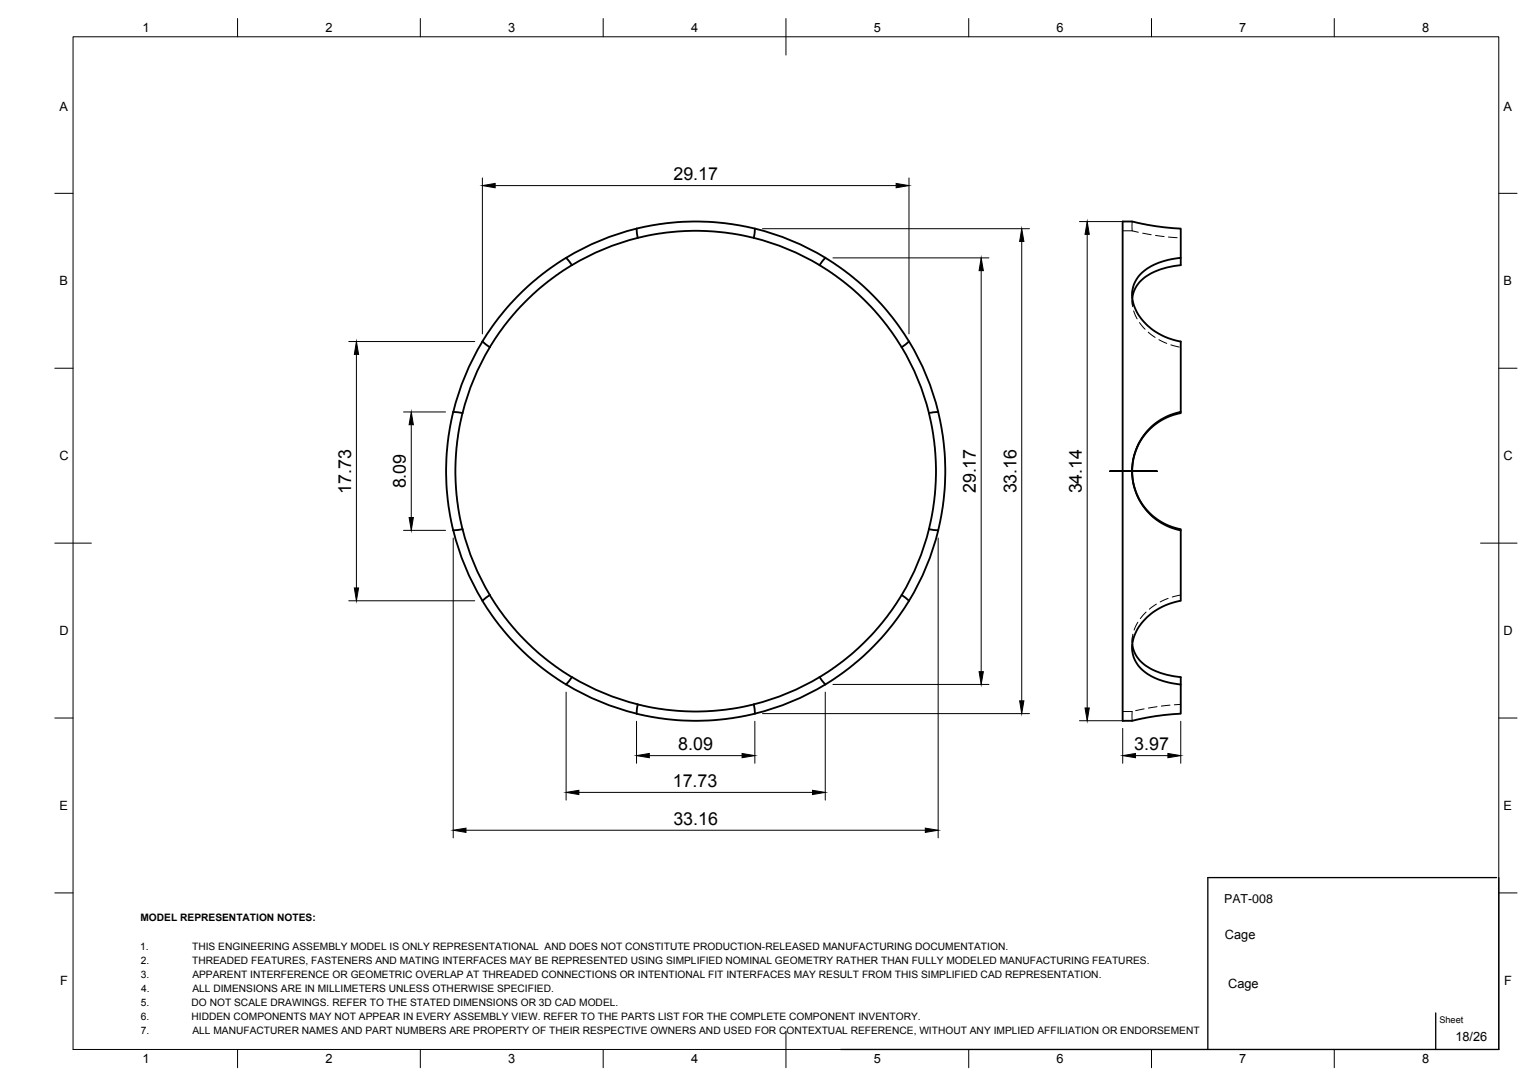
ISO-10303-21;
HEADER;
/* Generated by software containing ST-Developer
 * from STEP Tools, Inc. (www.steptools.com) 
 */

FILE_DESCRIPTION(
/* description */ ('Bearing housing with oil seal and end cap'),
/* implementation_level */ '2;1');

FILE_NAME(
/* name */ 'Cage.step',
/* time_stamp */ '2026-10-28T03:23:10-07:00',
/* author */ (''),
/* organization */ (''),
/* preprocessor_version */ 'ST-DEVELOPER v20.2',
/* originating_system */ 'Autodesk Translation Framework v15.17.0.0',
/* authorisation */ '');

FILE_SCHEMA (('AUTOMOTIVE_DESIGN { 1 0 10303 214 3 1 1 }'));
ENDSEC;

DATA;
#10=MECHANICAL_DESIGN_GEOMETRIC_PRESENTATION_REPRESENTATION('',(#277),#7871);
#159=B_SPLINE_CURVE_WITH_KNOTS('',3,(#6771,#6772,#6773,#6774,#6775,#6776,
#6777,#6778,#6779,#6780,#6781,#6782,#6783,#6784,#6785,#6786,#6787,#6788,
#6789,#6790,#6791,#6792),.UNSPECIFIED.,.F.,.F.,(4,2,2,2,2,2,2,2,2,2,4),
(0.0789094028588958,0.210573405340968,0.315860108011452,0.421146810681936,
0.522142632548711,0.623138454415485,0.72413427628226,0.825130098149035,
0.930416800819519,1.03570350349,1.16736750597208),.UNSPECIFIED.);
#160=B_SPLINE_CURVE_WITH_KNOTS('',3,(#6796,#6797,#6798,#6799,#6800,#6801,
#6802,#6803,#6804,#6805,#6806,#6807,#6808,#6809,#6810,#6811,#6812,#6813,
#6814,#6815,#6816,#6817),.UNSPECIFIED.,.F.,.F.,(4,2,2,2,2,2,2,2,2,2,4),
(0.0774793363974613,0.142088896491891,0.284177792983782,0.411119756996526,
0.514392970548519,0.617666184100513,0.720939397652506,0.8242126112045,0.951154575217244,
1.09324347170913,1.15785303180356),.UNSPECIFIED.);
#161=B_SPLINE_CURVE_WITH_KNOTS('',3,(#6823,#6824,#6825,#6826,#6827,#6828,
#6829,#6830,#6831,#6832,#6833,#6834,#6835,#6836,#6837,#6838,#6839,#6840,
#6841,#6842,#6843,#6844),.UNSPECIFIED.,.F.,.F.,(4,2,2,2,2,2,2,2,2,2,4),
(0.0774793363974613,0.142088896491891,0.284177792983782,0.411119756996525,
0.514392970548519,0.617666184100513,0.720939397652506,0.8242126112045,0.951154575217243,
1.09324347170913,1.15785303180356),.UNSPECIFIED.);
#162=B_SPLINE_CURVE_WITH_KNOTS('',3,(#6848,#6849,#6850,#6851,#6852,#6853,
#6854,#6855,#6856,#6857,#6858,#6859,#6860,#6861,#6862,#6863,#6864,#6865,
#6866,#6867,#6868,#6869),.UNSPECIFIED.,.F.,.F.,(4,2,2,2,2,2,2,2,2,2,4),
(0.0774793363974614,0.142088896491891,0.284177792983781,0.411119756996525,
0.514392970548519,0.617666184100512,0.720939397652506,0.824212611204499,
0.951154575217243,1.09324347170913,1.15785303180356),.UNSPECIFIED.);
#163=B_SPLINE_CURVE_WITH_KNOTS('',3,(#6873,#6874,#6875,#6876,#6877,#6878,
#6879,#6880,#6881,#6882,#6883,#6884),.UNSPECIFIED.,.F.,.F.,(4,2,2,2,2,4),
(0.0774793363974613,0.142088896491891,0.284177792983781,0.411119756996525,
0.514392970548519,0.617666184100512),.UNSPECIFIED.);
#164=B_SPLINE_CURVE_WITH_KNOTS('',3,(#6889,#6890,#6891,#6892,#6893,#6894,
#6895,#6896,#6897,#6898,#6899,#6900),.UNSPECIFIED.,.F.,.F.,(4,2,2,2,2,4),
(0.617666184100512,0.720939397652506,0.824212611204499,0.951154575217243,
1.09324347170913,1.15785303180356),.UNSPECIFIED.);
#165=B_SPLINE_CURVE_WITH_KNOTS('',3,(#6904,#6905,#6906,#6907,#6908,#6909,
#6910,#6911,#6912,#6913,#6914,#6915,#6916,#6917,#6918,#6919,#6920,#6921,
#6922,#6923,#6924,#6925),.UNSPECIFIED.,.F.,.F.,(4,2,2,2,2,2,2,2,2,2,4),
(0.0774793363974613,0.142088896491891,0.284177792983782,0.411119756996526,
0.514392970548519,0.617666184100513,0.720939397652507,0.8242126112045,0.951154575217245,
1.09324347170914,1.15785303180356),.UNSPECIFIED.);
#166=B_SPLINE_CURVE_WITH_KNOTS('',3,(#6929,#6930,#6931,#6932,#6933,#6934,
#6935,#6936,#6937,#6938,#6939,#6940,#6941,#6942,#6943,#6944,#6945,#6946,
#6947,#6948,#6949,#6950),.UNSPECIFIED.,.F.,.F.,(4,2,2,2,2,2,2,2,2,2,4),
(0.0774793363974613,0.142088896491891,0.284177792983782,0.411119756996526,
0.514392970548519,0.617666184100513,0.720939397652506,0.824212611204499,
0.951154575217243,1.09324347170913,1.15785303180356),.UNSPECIFIED.);
#167=B_SPLINE_CURVE_WITH_KNOTS('',3,(#6954,#6955,#6956,#6957,#6958,#6959,
#6960,#6961,#6962,#6963,#6964,#6965,#6966,#6967,#6968,#6969,#6970,#6971,
#6972,#6973,#6974,#6975),.UNSPECIFIED.,.F.,.F.,(4,2,2,2,2,2,2,2,2,2,4),
(0.0774793363974613,0.142088896491891,0.284177792983782,0.411119756996526,
0.514392970548519,0.617666184100513,0.720939397652506,0.8242126112045,0.951154575217244,
1.09324347170913,1.15785303180356),.UNSPECIFIED.);
#168=B_SPLINE_CURVE_WITH_KNOTS('',3,(#6979,#6980,#6981,#6982,#6983,#6984,
#6985,#6986,#6987,#6988,#6989,#6990,#6991,#6992,#6993,#6994,#6995,#6996,
#6997,#6998,#6999,#7000),.UNSPECIFIED.,.F.,.F.,(4,2,2,2,2,2,2,2,2,2,4),
(0.0774793363974613,0.142088896491891,0.284177792983782,0.411119756996526,
0.514392970548519,0.617666184100513,0.720939397652506,0.8242126112045,0.951154575217243,
1.09324347170913,1.15785303180356),.UNSPECIFIED.);
#169=B_SPLINE_CURVE_WITH_KNOTS('',3,(#7008,#7009,#7010,#7011,#7012,#7013,
#7014,#7015,#7016,#7017,#7018,#7019,#7020,#7021,#7022,#7023,#7024,#7025,
#7026,#7027,#7028,#7029),.UNSPECIFIED.,.F.,.F.,(4,2,2,2,2,2,2,2,2,2,4),
(0.0789094028588958,0.210573405340968,0.315860108011452,0.421146810681936,
0.522142632548711,0.623138454415485,0.72413427628226,0.825130098149035,
0.930416800819519,1.03570350349,1.16736750597208),.UNSPECIFIED.);
#170=B_SPLINE_CURVE_WITH_KNOTS('',3,(#7037,#7038,#7039,#7040,#7041,#7042,
#7043,#7044,#7045,#7046,#7047,#7048,#7049,#7050,#7051,#7052,#7053,#7054,
#7055,#7056,#7057,#7058),.UNSPECIFIED.,.F.,.F.,(4,2,2,2,2,2,2,2,2,2,4),
(0.0789094028588958,0.210573405340969,0.315860108011453,0.421146810681937,
0.522142632548712,0.623138454415486,0.724134276282261,0.825130098149035,
0.930416800819519,1.03570350349,1.16736750597208),.UNSPECIFIED.);
#171=B_SPLINE_CURVE_WITH_KNOTS('',3,(#7067,#7068,#7069,#7070,#7071,#7072,
#7073,#7074,#7075,#7076,#7077,#7078),.UNSPECIFIED.,.F.,.F.,(4,2,2,2,2,4),
(0.0789094028588958,0.210573405340968,0.315860108011452,0.421146810681937,
0.522142632548711,0.623138454415486),.UNSPECIFIED.);
#172=B_SPLINE_CURVE_WITH_KNOTS('',3,(#7080,#7081,#7082,#7083,#7084,#7085,
#7086,#7087,#7088,#7089,#7090,#7091),.UNSPECIFIED.,.F.,.F.,(4,2,2,2,2,4),
(0.623138454415486,0.72413427628226,0.825130098149035,0.930416800819519,
1.03570350349,1.16736750597208),.UNSPECIFIED.);
#173=B_SPLINE_CURVE_WITH_KNOTS('',3,(#7098,#7099,#7100,#7101,#7102,#7103,
#7104,#7105,#7106,#7107,#7108,#7109,#7110,#7111,#7112,#7113,#7114,#7115,
#7116,#7117,#7118,#7119),.UNSPECIFIED.,.F.,.F.,(4,2,2,2,2,2,2,2,2,2,4),
(0.0789094028588958,0.210573405340968,0.315860108011452,0.421146810681936,
0.522142632548711,0.623138454415486,0.72413427628226,0.825130098149035,
0.930416800819519,1.03570350349,1.16736750597208),.UNSPECIFIED.);
#174=B_SPLINE_CURVE_WITH_KNOTS('',3,(#7127,#7128,#7129,#7130,#7131,#7132,
#7133,#7134,#7135,#7136,#7137,#7138,#7139,#7140,#7141,#7142,#7143,#7144,
#7145,#7146,#7147,#7148),.UNSPECIFIED.,.F.,.F.,(4,2,2,2,2,2,2,2,2,2,4),
(0.0789094028588957,0.210573405340968,0.315860108011452,0.421146810681936,
0.522142632548711,0.623138454415485,0.72413427628226,0.825130098149035,
0.930416800819519,1.03570350349,1.16736750597207),.UNSPECIFIED.);
#175=B_SPLINE_CURVE_WITH_KNOTS('',3,(#7156,#7157,#7158,#7159,#7160,#7161,
#7162,#7163,#7164,#7165,#7166,#7167,#7168,#7169,#7170,#7171,#7172,#7173,
#7174,#7175,#7176,#7177),.UNSPECIFIED.,.F.,.F.,(4,2,2,2,2,2,2,2,2,2,4),
(0.0789094028588958,0.210573405340968,0.315860108011452,0.421146810681936,
0.522142632548711,0.623138454415486,0.72413427628226,0.825130098149035,
0.930416800819519,1.03570350349,1.16736750597208),.UNSPECIFIED.);
#176=B_SPLINE_CURVE_WITH_KNOTS('',3,(#7186,#7187,#7188,#7189,#7190,#7191,
#7192,#7193,#7194,#7195,#7196,#7197,#7198,#7199,#7200,#7201,#7202,#7203,
#7204,#7205,#7206,#7207),.UNSPECIFIED.,.F.,.F.,(4,2,2,2,2,2,2,2,2,2,4),
(0.0789094028588958,0.210573405340968,0.315860108011452,0.421146810681936,
0.522142632548711,0.623138454415485,0.72413427628226,0.825130098149035,
0.930416800819519,1.03570350349,1.16736750597208),.UNSPECIFIED.);
#193=SPHERICAL_SURFACE('',#4614,0.412776);
#194=SPHERICAL_SURFACE('',#4630,0.412776);
#195=SPHERICAL_SURFACE('',#4635,0.412776);
#196=SPHERICAL_SURFACE('',#4640,0.412776);
#197=SPHERICAL_SURFACE('',#4645,0.412776);
#198=SPHERICAL_SURFACE('',#4650,0.412776);
#199=SPHERICAL_SURFACE('',#4655,0.412776);
#200=SPHERICAL_SURFACE('',#4663,0.412776);
#228=SHAPE_REPRESENTATION_RELATIONSHIP('SRR','None',#7976,#249);
#249=ADVANCED_BREP_SHAPE_REPRESENTATION('',(#306),#7860);
#277=STYLED_ITEM('',(#8153),#306);
#306=MANIFOLD_SOLID_BREP('Continuous crown cage',#4103);
#378=FACE_BOUND('',#1013,.T.);
#475=PLANE('',#4627);
#476=PLANE('',#4632);
#477=PLANE('',#4637);
#478=PLANE('',#4642);
#479=PLANE('',#4647);
#480=PLANE('',#4652);
#481=PLANE('',#4661);
#482=PLANE('',#4665);
#483=PLANE('',#4666);
#681=FACE_OUTER_BOUND('',#995,.T.);
#682=FACE_OUTER_BOUND('',#996,.T.);
#683=FACE_OUTER_BOUND('',#997,.T.);
#684=FACE_OUTER_BOUND('',#998,.T.);
#685=FACE_OUTER_BOUND('',#999,.T.);
#686=FACE_OUTER_BOUND('',#1000,.T.);
#687=FACE_OUTER_BOUND('',#1001,.T.);
#688=FACE_OUTER_BOUND('',#1002,.T.);
#689=FACE_OUTER_BOUND('',#1003,.T.);
#690=FACE_OUTER_BOUND('',#1004,.T.);
#691=FACE_OUTER_BOUND('',#1005,.T.);
#692=FACE_OUTER_BOUND('',#1006,.T.);
#693=FACE_OUTER_BOUND('',#1007,.T.);
#694=FACE_OUTER_BOUND('',#1008,.T.);
#695=FACE_OUTER_BOUND('',#1009,.T.);
#696=FACE_OUTER_BOUND('',#1010,.T.);
#697=FACE_OUTER_BOUND('',#1011,.T.);
#698=FACE_OUTER_BOUND('',#1012,.T.);
#699=FACE_OUTER_BOUND('',#1014,.T.);
#995=EDGE_LOOP('',(#3235,#3236,#3237,#3238));
#996=EDGE_LOOP('',(#3239,#3240,#3241,#3242,#3243,#3244,#3245,#3246,#3247,
#3248,#3249,#3250,#3251,#3252,#3253,#3254,#3255,#3256,#3257,#3258));
#997=EDGE_LOOP('',(#3259,#3260,#3261,#3262));
#998=EDGE_LOOP('',(#3263,#3264,#3265,#3266));
#999=EDGE_LOOP('',(#3267,#3268,#3269,#3270));
#1000=EDGE_LOOP('',(#3271,#3272,#3273,#3274));
#1001=EDGE_LOOP('',(#3275,#3276,#3277,#3278));
#1002=EDGE_LOOP('',(#3279,#3280,#3281,#3282,#3283,#3284));
#1003=EDGE_LOOP('',(#3285,#3286,#3287,#3288));
#1004=EDGE_LOOP('',(#3289,#3290,#3291,#3292));
#1005=EDGE_LOOP('',(#3293,#3294,#3295,#3296));
#1006=EDGE_LOOP('',(#3297,#3298,#3299,#3300));
#1007=EDGE_LOOP('',(#3301,#3302,#3303,#3304));
#1008=EDGE_LOOP('',(#3305,#3306,#3307,#3308));
#1009=EDGE_LOOP('',(#3309,#3310,#3311,#3312,#3313,#3314,#3315,#3316,#3317,
#3318,#3319,#3320,#3321,#3322,#3323,#3324,#3325,#3326,#3327,#3328));
#1010=EDGE_LOOP('',(#3329,#3330,#3331,#3332));
#1011=EDGE_LOOP('',(#3333,#3334,#3335,#3336));
#1012=EDGE_LOOP('',(#3337));
#1013=EDGE_LOOP('',(#3338));
#1014=EDGE_LOOP('',(#3339,#3340,#3341,#3342));
#1271=LINE('',#6886,#1533);
#1272=LINE('',#7182,#1534);
#1533=VECTOR('',#5550,1.706752);
#1534=VECTOR('',#5627,1.643248);
#1793=CIRCLE('',#4615,0.405071403305639);
#1794=CIRCLE('',#4616,0.405071403305639);
#1795=CIRCLE('',#4618,1.706752);
#1796=CIRCLE('',#4619,1.706752);
#1797=CIRCLE('',#4620,1.706752);
#1798=CIRCLE('',#4621,1.706752);
#1799=CIRCLE('',#4622,1.706752);
#1800=CIRCLE('',#4623,1.706752);
#1801=CIRCLE('',#4624,1.706752);
#1802=CIRCLE('',#4625,1.706752);
#1803=CIRCLE('',#4626,1.706752);
#1804=CIRCLE('',#4628,1.643248);
#1805=CIRCLE('',#4629,0.405071403305639);
#1806=CIRCLE('',#4631,0.405071403305639);
#1807=CIRCLE('',#4633,1.643248);
#1808=CIRCLE('',#4634,0.405071403305639);
#1809=CIRCLE('',#4636,0.405071403305639);
#1810=CIRCLE('',#4638,1.643248);
#1811=CIRCLE('',#4639,0.405071403305639);
#1812=CIRCLE('',#4641,0.405071403305639);
#1813=CIRCLE('',#4643,1.643248);
#1814=CIRCLE('',#4644,0.405071403305639);
#1815=CIRCLE('',#4646,0.405071403305639);
#1816=CIRCLE('',#4648,1.643248);
#1817=CIRCLE('',#4649,0.405071403305639);
#1818=CIRCLE('',#4651,0.405071403305639);
#1819=CIRCLE('',#4653,1.643248);
#1820=CIRCLE('',#4654,0.405071403305639);
#1821=CIRCLE('',#4656,0.405071403305639);
#1822=CIRCLE('',#4658,1.643248);
#1823=CIRCLE('',#4659,1.643248);
#1824=CIRCLE('',#4660,1.643248);
#1825=CIRCLE('',#4662,0.405071403305639);
#1826=CIRCLE('',#4664,0.405071403305639);
#2063=VERTEX_POINT('',#6769);
#2064=VERTEX_POINT('',#6770);
#2065=VERTEX_POINT('',#6793);
#2066=VERTEX_POINT('',#6795);
#2067=VERTEX_POINT('',#6820);
#2068=VERTEX_POINT('',#6822);
#2069=VERTEX_POINT('',#6845);
#2070=VERTEX_POINT('',#6847);
#2071=VERTEX_POINT('',#6870);
#2072=VERTEX_POINT('',#6872);
#2073=VERTEX_POINT('',#6885);
#2074=VERTEX_POINT('',#6888);
#2075=VERTEX_POINT('',#6901);
#2076=VERTEX_POINT('',#6903);
#2077=VERTEX_POINT('',#6926);
#2078=VERTEX_POINT('',#6928);
#2079=VERTEX_POINT('',#6951);
#2080=VERTEX_POINT('',#6953);
#2081=VERTEX_POINT('',#6976);
#2082=VERTEX_POINT('',#6978);
#2083=VERTEX_POINT('',#7003);
#2084=VERTEX_POINT('',#7007);
#2085=VERTEX_POINT('',#7032);
#2086=VERTEX_POINT('',#7036);
#2087=VERTEX_POINT('',#7061);
#2088=VERTEX_POINT('',#7065);
#2089=VERTEX_POINT('',#7066);
#2090=VERTEX_POINT('',#7093);
#2091=VERTEX_POINT('',#7097);
#2092=VERTEX_POINT('',#7122);
#2093=VERTEX_POINT('',#7126);
#2094=VERTEX_POINT('',#7151);
#2095=VERTEX_POINT('',#7155);
#2096=VERTEX_POINT('',#7180);
#2097=VERTEX_POINT('',#7183);
#2098=VERTEX_POINT('',#7185);
#2481=EDGE_CURVE('',#2063,#2064,#159,.T.);
#2482=EDGE_CURVE('',#2065,#2063,#1793,.T.);
#2483=EDGE_CURVE('',#2066,#2065,#160,.T.);
#2484=EDGE_CURVE('',#2064,#2066,#1794,.T.);
#2485=EDGE_CURVE('',#2067,#2065,#1795,.T.);
#2486=EDGE_CURVE('',#2067,#2068,#161,.T.);
#2487=EDGE_CURVE('',#2069,#2068,#1796,.T.);
#2488=EDGE_CURVE('',#2069,#2070,#162,.T.);
#2489=EDGE_CURVE('',#2071,#2070,#1797,.T.);
#2490=EDGE_CURVE('',#2071,#2072,#163,.T.);
#2491=EDGE_CURVE('',#2072,#2073,#1271,.T.);
#2492=EDGE_CURVE('',#2073,#2073,#1798,.T.);
#2493=EDGE_CURVE('',#2072,#2074,#164,.T.);
#2494=EDGE_CURVE('',#2075,#2074,#1799,.T.);
#2495=EDGE_CURVE('',#2075,#2076,#165,.T.);
#2496=EDGE_CURVE('',#2077,#2076,#1800,.T.);
#2497=EDGE_CURVE('',#2077,#2078,#166,.T.);
#2498=EDGE_CURVE('',#2079,#2078,#1801,.T.);
#2499=EDGE_CURVE('',#2079,#2080,#167,.T.);
#2500=EDGE_CURVE('',#2081,#2080,#1802,.T.);
#2501=EDGE_CURVE('',#2081,#2082,#168,.T.);
#2502=EDGE_CURVE('',#2066,#2082,#1803,.T.);
#2503=EDGE_CURVE('',#2063,#2083,#1804,.T.);
#2504=EDGE_CURVE('',#2083,#2067,#1805,.T.);
#2505=EDGE_CURVE('',#2084,#2083,#169,.T.);
#2506=EDGE_CURVE('',#2068,#2084,#1806,.T.);
#2507=EDGE_CURVE('',#2084,#2085,#1807,.T.);
#2508=EDGE_CURVE('',#2085,#2069,#1808,.T.);
#2509=EDGE_CURVE('',#2086,#2085,#170,.T.);
#2510=EDGE_CURVE('',#2070,#2086,#1809,.T.);
#2511=EDGE_CURVE('',#2086,#2087,#1810,.T.);
#2512=EDGE_CURVE('',#2087,#2071,#1811,.T.);
#2513=EDGE_CURVE('',#2088,#2089,#171,.T.);
#2514=EDGE_CURVE('',#2074,#2088,#1812,.T.);
#2515=EDGE_CURVE('',#2089,#2087,#172,.T.);
#2516=EDGE_CURVE('',#2088,#2090,#1813,.T.);
#2517=EDGE_CURVE('',#2090,#2075,#1814,.T.);
#2518=EDGE_CURVE('',#2091,#2090,#173,.T.);
#2519=EDGE_CURVE('',#2076,#2091,#1815,.T.);
#2520=EDGE_CURVE('',#2091,#2092,#1816,.T.);
#2521=EDGE_CURVE('',#2092,#2077,#1817,.T.);
#2522=EDGE_CURVE('',#2093,#2092,#174,.T.);
#2523=EDGE_CURVE('',#2078,#2093,#1818,.T.);
#2524=EDGE_CURVE('',#2093,#2094,#1819,.T.);
#2525=EDGE_CURVE('',#2094,#2079,#1820,.T.);
#2526=EDGE_CURVE('',#2095,#2094,#175,.T.);
#2527=EDGE_CURVE('',#2080,#2095,#1821,.T.);
#2528=EDGE_CURVE('',#2096,#2096,#1822,.T.);
#2529=EDGE_CURVE('',#2096,#2089,#1272,.T.);
#2530=EDGE_CURVE('',#2097,#2064,#1823,.T.);
#2531=EDGE_CURVE('',#2097,#2098,#176,.T.);
#2532=EDGE_CURVE('',#2095,#2098,#1824,.T.);
#2533=EDGE_CURVE('',#2082,#2097,#1825,.T.);
#2534=EDGE_CURVE('',#2098,#2081,#1826,.T.);
#3235=ORIENTED_EDGE('',*,*,#2481,.F.);
#3236=ORIENTED_EDGE('',*,*,#2482,.F.);
#3237=ORIENTED_EDGE('',*,*,#2483,.F.);
#3238=ORIENTED_EDGE('',*,*,#2484,.F.);
#3239=ORIENTED_EDGE('',*,*,#2483,.T.);
#3240=ORIENTED_EDGE('',*,*,#2485,.F.);
#3241=ORIENTED_EDGE('',*,*,#2486,.T.);
#3242=ORIENTED_EDGE('',*,*,#2487,.F.);
#3243=ORIENTED_EDGE('',*,*,#2488,.T.);
#3244=ORIENTED_EDGE('',*,*,#2489,.F.);
#3245=ORIENTED_EDGE('',*,*,#2490,.T.);
#3246=ORIENTED_EDGE('',*,*,#2491,.T.);
#3247=ORIENTED_EDGE('',*,*,#2492,.F.);
#3248=ORIENTED_EDGE('',*,*,#2491,.F.);
#3249=ORIENTED_EDGE('',*,*,#2493,.T.);
#3250=ORIENTED_EDGE('',*,*,#2494,.F.);
#3251=ORIENTED_EDGE('',*,*,#2495,.T.);
#3252=ORIENTED_EDGE('',*,*,#2496,.F.);
#3253=ORIENTED_EDGE('',*,*,#2497,.T.);
#3254=ORIENTED_EDGE('',*,*,#2498,.F.);
#3255=ORIENTED_EDGE('',*,*,#2499,.T.);
#3256=ORIENTED_EDGE('',*,*,#2500,.F.);
#3257=ORIENTED_EDGE('',*,*,#2501,.T.);
#3258=ORIENTED_EDGE('',*,*,#2502,.F.);
#3259=ORIENTED_EDGE('',*,*,#2482,.T.);
#3260=ORIENTED_EDGE('',*,*,#2503,.T.);
#3261=ORIENTED_EDGE('',*,*,#2504,.T.);
#3262=ORIENTED_EDGE('',*,*,#2485,.T.);
#3263=ORIENTED_EDGE('',*,*,#2505,.F.);
#3264=ORIENTED_EDGE('',*,*,#2506,.F.);
#3265=ORIENTED_EDGE('',*,*,#2486,.F.);
#3266=ORIENTED_EDGE('',*,*,#2504,.F.);
#3267=ORIENTED_EDGE('',*,*,#2506,.T.);
#3268=ORIENTED_EDGE('',*,*,#2507,.T.);
#3269=ORIENTED_EDGE('',*,*,#2508,.T.);
#3270=ORIENTED_EDGE('',*,*,#2487,.T.);
#3271=ORIENTED_EDGE('',*,*,#2509,.F.);
#3272=ORIENTED_EDGE('',*,*,#2510,.F.);
#3273=ORIENTED_EDGE('',*,*,#2488,.F.);
#3274=ORIENTED_EDGE('',*,*,#2508,.F.);
#3275=ORIENTED_EDGE('',*,*,#2510,.T.);
#3276=ORIENTED_EDGE('',*,*,#2511,.T.);
#3277=ORIENTED_EDGE('',*,*,#2512,.T.);
#3278=ORIENTED_EDGE('',*,*,#2489,.T.);
#3279=ORIENTED_EDGE('',*,*,#2513,.F.);
#3280=ORIENTED_EDGE('',*,*,#2514,.F.);
#3281=ORIENTED_EDGE('',*,*,#2493,.F.);
#3282=ORIENTED_EDGE('',*,*,#2490,.F.);
#3283=ORIENTED_EDGE('',*,*,#2512,.F.);
#3284=ORIENTED_EDGE('',*,*,#2515,.F.);
#3285=ORIENTED_EDGE('',*,*,#2514,.T.);
#3286=ORIENTED_EDGE('',*,*,#2516,.T.);
#3287=ORIENTED_EDGE('',*,*,#2517,.T.);
#3288=ORIENTED_EDGE('',*,*,#2494,.T.);
#3289=ORIENTED_EDGE('',*,*,#2518,.F.);
#3290=ORIENTED_EDGE('',*,*,#2519,.F.);
#3291=ORIENTED_EDGE('',*,*,#2495,.F.);
#3292=ORIENTED_EDGE('',*,*,#2517,.F.);
#3293=ORIENTED_EDGE('',*,*,#2519,.T.);
#3294=ORIENTED_EDGE('',*,*,#2520,.T.);
#3295=ORIENTED_EDGE('',*,*,#2521,.T.);
#3296=ORIENTED_EDGE('',*,*,#2496,.T.);
#3297=ORIENTED_EDGE('',*,*,#2522,.F.);
#3298=ORIENTED_EDGE('',*,*,#2523,.F.);
#3299=ORIENTED_EDGE('',*,*,#2497,.F.);
#3300=ORIENTED_EDGE('',*,*,#2521,.F.);
#3301=ORIENTED_EDGE('',*,*,#2523,.T.);
#3302=ORIENTED_EDGE('',*,*,#2524,.T.);
#3303=ORIENTED_EDGE('',*,*,#2525,.T.);
#3304=ORIENTED_EDGE('',*,*,#2498,.T.);
#3305=ORIENTED_EDGE('',*,*,#2499,.F.);
#3306=ORIENTED_EDGE('',*,*,#2525,.F.);
#3307=ORIENTED_EDGE('',*,*,#2526,.F.);
#3308=ORIENTED_EDGE('',*,*,#2527,.F.);
#3309=ORIENTED_EDGE('',*,*,#2528,.F.);
#3310=ORIENTED_EDGE('',*,*,#2529,.T.);
#3311=ORIENTED_EDGE('',*,*,#2515,.T.);
#3312=ORIENTED_EDGE('',*,*,#2511,.F.);
#3313=ORIENTED_EDGE('',*,*,#2509,.T.);
#3314=ORIENTED_EDGE('',*,*,#2507,.F.);
#3315=ORIENTED_EDGE('',*,*,#2505,.T.);
#3316=ORIENTED_EDGE('',*,*,#2503,.F.);
#3317=ORIENTED_EDGE('',*,*,#2481,.T.);
#3318=ORIENTED_EDGE('',*,*,#2530,.F.);
#3319=ORIENTED_EDGE('',*,*,#2531,.T.);
#3320=ORIENTED_EDGE('',*,*,#2532,.F.);
#3321=ORIENTED_EDGE('',*,*,#2526,.T.);
#3322=ORIENTED_EDGE('',*,*,#2524,.F.);
#3323=ORIENTED_EDGE('',*,*,#2522,.T.);
#3324=ORIENTED_EDGE('',*,*,#2520,.F.);
#3325=ORIENTED_EDGE('',*,*,#2518,.T.);
#3326=ORIENTED_EDGE('',*,*,#2516,.F.);
#3327=ORIENTED_EDGE('',*,*,#2513,.T.);
#3328=ORIENTED_EDGE('',*,*,#2529,.F.);
#3329=ORIENTED_EDGE('',*,*,#2484,.T.);
#3330=ORIENTED_EDGE('',*,*,#2502,.T.);
#3331=ORIENTED_EDGE('',*,*,#2533,.T.);
#3332=ORIENTED_EDGE('',*,*,#2530,.T.);
#3333=ORIENTED_EDGE('',*,*,#2501,.F.);
#3334=ORIENTED_EDGE('',*,*,#2534,.F.);
#3335=ORIENTED_EDGE('',*,*,#2531,.F.);
#3336=ORIENTED_EDGE('',*,*,#2533,.F.);
#3337=ORIENTED_EDGE('',*,*,#2492,.T.);
#3338=ORIENTED_EDGE('',*,*,#2528,.T.);
#3339=ORIENTED_EDGE('',*,*,#2527,.T.);
#3340=ORIENTED_EDGE('',*,*,#2532,.T.);
#3341=ORIENTED_EDGE('',*,*,#2534,.T.);
#3342=ORIENTED_EDGE('',*,*,#2500,.T.);
#3807=CYLINDRICAL_SURFACE('',#4617,1.706752);
#3808=CYLINDRICAL_SURFACE('',#4657,1.643248);
#3963=ADVANCED_FACE('',(#681),#193,.F.);
#3964=ADVANCED_FACE('',(#682),#3807,.T.);
#3965=ADVANCED_FACE('',(#683),#475,.T.);
#3966=ADVANCED_FACE('',(#684),#194,.F.);
#3967=ADVANCED_FACE('',(#685),#476,.T.);
#3968=ADVANCED_FACE('',(#686),#195,.F.);
#3969=ADVANCED_FACE('',(#687),#477,.T.);
#3970=ADVANCED_FACE('',(#688),#196,.F.);
#3971=ADVANCED_FACE('',(#689),#478,.T.);
#3972=ADVANCED_FACE('',(#690),#197,.F.);
#3973=ADVANCED_FACE('',(#691),#479,.T.);
#3974=ADVANCED_FACE('',(#692),#198,.F.);
#3975=ADVANCED_FACE('',(#693),#480,.T.);
#3976=ADVANCED_FACE('',(#694),#199,.F.);
#3977=ADVANCED_FACE('',(#695),#3808,.F.);
#3978=ADVANCED_FACE('',(#696),#481,.T.);
#3979=ADVANCED_FACE('',(#697),#200,.F.);
#3980=ADVANCED_FACE('',(#698,#378),#482,.T.);
#3981=ADVANCED_FACE('',(#699),#483,.T.);
#4103=CLOSED_SHELL('',(#3963,#3964,#3965,#3966,#3967,#3968,#3969,#3970,
#3971,#3972,#3973,#3974,#3975,#3976,#3977,#3978,#3979,#3980,#3981));
#4613=AXIS2_PLACEMENT_3D('',#6767,#5534,#5535);
#4614=AXIS2_PLACEMENT_3D('',#6768,#5536,#5537);
#4615=AXIS2_PLACEMENT_3D('',#6794,#5538,#5539);
#4616=AXIS2_PLACEMENT_3D('',#6818,#5540,#5541);
#4617=AXIS2_PLACEMENT_3D('',#6819,#5542,#5543);
#4618=AXIS2_PLACEMENT_3D('',#6821,#5544,#5545);
#4619=AXIS2_PLACEMENT_3D('',#6846,#5546,#5547);
#4620=AXIS2_PLACEMENT_3D('',#6871,#5548,#5549);
#4621=AXIS2_PLACEMENT_3D('',#6887,#5551,#5552);
#4622=AXIS2_PLACEMENT_3D('',#6902,#5553,#5554);
#4623=AXIS2_PLACEMENT_3D('',#6927,#5555,#5556);
#4624=AXIS2_PLACEMENT_3D('',#6952,#5557,#5558);
#4625=AXIS2_PLACEMENT_3D('',#6977,#5559,#5560);
#4626=AXIS2_PLACEMENT_3D('',#7001,#5561,#5562);
#4627=AXIS2_PLACEMENT_3D('',#7002,#5563,#5564);
#4628=AXIS2_PLACEMENT_3D('',#7004,#5565,#5566);
#4629=AXIS2_PLACEMENT_3D('',#7005,#5567,#5568);
#4630=AXIS2_PLACEMENT_3D('',#7006,#5569,#5570);
#4631=AXIS2_PLACEMENT_3D('',#7030,#5571,#5572);
#4632=AXIS2_PLACEMENT_3D('',#7031,#5573,#5574);
#4633=AXIS2_PLACEMENT_3D('',#7033,#5575,#5576);
#4634=AXIS2_PLACEMENT_3D('',#7034,#5577,#5578);
#4635=AXIS2_PLACEMENT_3D('',#7035,#5579,#5580);
#4636=AXIS2_PLACEMENT_3D('',#7059,#5581,#5582);
#4637=AXIS2_PLACEMENT_3D('',#7060,#5583,#5584);
#4638=AXIS2_PLACEMENT_3D('',#7062,#5585,#5586);
#4639=AXIS2_PLACEMENT_3D('',#7063,#5587,#5588);
#4640=AXIS2_PLACEMENT_3D('',#7064,#5589,#5590);
#4641=AXIS2_PLACEMENT_3D('',#7079,#5591,#5592);
#4642=AXIS2_PLACEMENT_3D('',#7092,#5593,#5594);
#4643=AXIS2_PLACEMENT_3D('',#7094,#5595,#5596);
#4644=AXIS2_PLACEMENT_3D('',#7095,#5597,#5598);
#4645=AXIS2_PLACEMENT_3D('',#7096,#5599,#5600);
#4646=AXIS2_PLACEMENT_3D('',#7120,#5601,#5602);
#4647=AXIS2_PLACEMENT_3D('',#7121,#5603,#5604);
#4648=AXIS2_PLACEMENT_3D('',#7123,#5605,#5606);
#4649=AXIS2_PLACEMENT_3D('',#7124,#5607,#5608);
#4650=AXIS2_PLACEMENT_3D('',#7125,#5609,#5610);
#4651=AXIS2_PLACEMENT_3D('',#7149,#5611,#5612);
#4652=AXIS2_PLACEMENT_3D('',#7150,#5613,#5614);
#4653=AXIS2_PLACEMENT_3D('',#7152,#5615,#5616);
#4654=AXIS2_PLACEMENT_3D('',#7153,#5617,#5618);
#4655=AXIS2_PLACEMENT_3D('',#7154,#5619,#5620);
#4656=AXIS2_PLACEMENT_3D('',#7178,#5621,#5622);
#4657=AXIS2_PLACEMENT_3D('',#7179,#5623,#5624);
#4658=AXIS2_PLACEMENT_3D('',#7181,#5625,#5626);
#4659=AXIS2_PLACEMENT_3D('',#7184,#5628,#5629);
#4660=AXIS2_PLACEMENT_3D('',#7208,#5630,#5631);
#4661=AXIS2_PLACEMENT_3D('',#7209,#5632,#5633);
#4662=AXIS2_PLACEMENT_3D('',#7210,#5634,#5635);
#4663=AXIS2_PLACEMENT_3D('',#7211,#5636,#5637);
#4664=AXIS2_PLACEMENT_3D('',#7212,#5638,#5639);
#4665=AXIS2_PLACEMENT_3D('',#7213,#5640,#5641);
#4666=AXIS2_PLACEMENT_3D('',#7214,#5642,#5643);
#5534=DIRECTION('axis',(0.,0.,1.));
#5535=DIRECTION('refdir',(1.,0.,0.));
#5536=DIRECTION('center_axis',(0.,0.,1.));
#5537=DIRECTION('ref_axis',(1.,0.,0.));
#5538=DIRECTION('center_axis',(0.,-1.,0.));
#5539=DIRECTION('ref_axis',(0.,0.,-1.));
#5540=DIRECTION('center_axis',(0.,-1.,0.));
#5541=DIRECTION('ref_axis',(0.,0.,-1.));
#5542=DIRECTION('center_axis',(0.,1.,0.));
#5543=DIRECTION('ref_axis',(1.,0.,0.));
#5544=DIRECTION('center_axis',(0.,1.,0.));
#5545=DIRECTION('ref_axis',(1.,0.,0.));
#5546=DIRECTION('center_axis',(0.,1.,0.));
#5547=DIRECTION('ref_axis',(1.,0.,0.));
#5548=DIRECTION('center_axis',(0.,1.,0.));
#5549=DIRECTION('ref_axis',(1.,0.,0.));
#5550=DIRECTION('',(0.,-1.,0.));
#5551=DIRECTION('center_axis',(0.,-1.,0.));
#5552=DIRECTION('ref_axis',(1.,0.,0.));
#5553=DIRECTION('center_axis',(0.,1.,0.));
#5554=DIRECTION('ref_axis',(1.,0.,0.));
#5555=DIRECTION('center_axis',(0.,1.,0.));
#5556=DIRECTION('ref_axis',(1.,0.,0.));
#5557=DIRECTION('center_axis',(0.,1.,0.));
#5558=DIRECTION('ref_axis',(1.,0.,0.));
#5559=DIRECTION('center_axis',(0.,1.,0.));
#5560=DIRECTION('ref_axis',(1.,0.,0.));
#5561=DIRECTION('center_axis',(0.,1.,0.));
#5562=DIRECTION('ref_axis',(1.,0.,0.));
#5563=DIRECTION('center_axis',(0.,1.,0.));
#5564=DIRECTION('ref_axis',(1.,0.,0.));
#5565=DIRECTION('center_axis',(0.,-1.,0.));
#5566=DIRECTION('ref_axis',(1.,0.,0.));
#5567=DIRECTION('center_axis',(0.,-1.,0.));
#5568=DIRECTION('ref_axis',(0.,0.,-1.));
#5569=DIRECTION('center_axis',(6.12323399573677E-17,0.,1.));
#5570=DIRECTION('ref_axis',(1.,0.,0.));
#5571=DIRECTION('center_axis',(0.,-1.,0.));
#5572=DIRECTION('ref_axis',(0.,0.,-1.));
#5573=DIRECTION('center_axis',(0.,1.,0.));
#5574=DIRECTION('ref_axis',(1.,0.,0.));
#5575=DIRECTION('center_axis',(0.,-1.,0.));
#5576=DIRECTION('ref_axis',(1.,0.,0.));
#5577=DIRECTION('center_axis',(0.,-1.,0.));
#5578=DIRECTION('ref_axis',(0.,0.,-1.));
#5579=DIRECTION('center_axis',(0.,0.,1.));
#5580=DIRECTION('ref_axis',(1.,0.,0.));
#5581=DIRECTION('center_axis',(0.,-1.,0.));
#5582=DIRECTION('ref_axis',(0.,0.,-1.));
#5583=DIRECTION('center_axis',(0.,1.,0.));
#5584=DIRECTION('ref_axis',(1.,0.,0.));
#5585=DIRECTION('center_axis',(0.,-1.,0.));
#5586=DIRECTION('ref_axis',(1.,0.,0.));
#5587=DIRECTION('center_axis',(0.,-1.,0.));
#5588=DIRECTION('ref_axis',(0.,0.,-1.));
#5589=DIRECTION('center_axis',(0.,0.,1.));
#5590=DIRECTION('ref_axis',(1.,0.,0.));
#5591=DIRECTION('center_axis',(0.,-1.,0.));
#5592=DIRECTION('ref_axis',(0.,0.,-1.));
#5593=DIRECTION('center_axis',(0.,1.,0.));
#5594=DIRECTION('ref_axis',(1.,0.,0.));
#5595=DIRECTION('center_axis',(0.,-1.,0.));
#5596=DIRECTION('ref_axis',(1.,0.,0.));
#5597=DIRECTION('center_axis',(0.,-1.,0.));
#5598=DIRECTION('ref_axis',(0.,0.,-1.));
#5599=DIRECTION('center_axis',(0.,0.,1.));
#5600=DIRECTION('ref_axis',(1.,0.,0.));
#5601=DIRECTION('center_axis',(0.,-1.,0.));
#5602=DIRECTION('ref_axis',(0.,0.,-1.));
#5603=DIRECTION('center_axis',(0.,1.,0.));
#5604=DIRECTION('ref_axis',(1.,0.,0.));
#5605=DIRECTION('center_axis',(0.,-1.,0.));
#5606=DIRECTION('ref_axis',(1.,0.,0.));
#5607=DIRECTION('center_axis',(0.,-1.,0.));
#5608=DIRECTION('ref_axis',(0.,0.,-1.));
#5609=DIRECTION('center_axis',(6.12323399573676E-17,0.,1.));
#5610=DIRECTION('ref_axis',(1.,0.,0.));
#5611=DIRECTION('center_axis',(0.,-1.,0.));
#5612=DIRECTION('ref_axis',(0.,0.,-1.));
#5613=DIRECTION('center_axis',(0.,1.,0.));
#5614=DIRECTION('ref_axis',(1.,0.,0.));
#5615=DIRECTION('center_axis',(0.,-1.,0.));
#5616=DIRECTION('ref_axis',(1.,0.,0.));
#5617=DIRECTION('center_axis',(0.,-1.,0.));
#5618=DIRECTION('ref_axis',(0.,0.,-1.));
#5619=DIRECTION('center_axis',(0.,0.,1.));
#5620=DIRECTION('ref_axis',(1.,0.,0.));
#5621=DIRECTION('center_axis',(0.,-1.,0.));
#5622=DIRECTION('ref_axis',(0.,0.,-1.));
#5623=DIRECTION('center_axis',(0.,1.,0.));
#5624=DIRECTION('ref_axis',(1.,0.,0.));
#5625=DIRECTION('center_axis',(0.,1.,0.));
#5626=DIRECTION('ref_axis',(1.,0.,0.));
#5627=DIRECTION('',(0.,1.,0.));
#5628=DIRECTION('center_axis',(0.,-1.,0.));
#5629=DIRECTION('ref_axis',(1.,0.,0.));
#5630=DIRECTION('center_axis',(0.,-1.,0.));
#5631=DIRECTION('ref_axis',(1.,0.,0.));
#5632=DIRECTION('center_axis',(0.,1.,0.));
#5633=DIRECTION('ref_axis',(1.,0.,0.));
#5634=DIRECTION('center_axis',(0.,-1.,0.));
#5635=DIRECTION('ref_axis',(0.,0.,-1.));
#5636=DIRECTION('center_axis',(0.,0.,1.));
#5637=DIRECTION('ref_axis',(1.,0.,0.));
#5638=DIRECTION('center_axis',(0.,-1.,0.));
#5639=DIRECTION('ref_axis',(0.,0.,-1.));
#5640=DIRECTION('center_axis',(0.,-1.,0.));
#5641=DIRECTION('ref_axis',(-1.,0.,0.));
#5642=DIRECTION('center_axis',(0.,1.,0.));
#5643=DIRECTION('ref_axis',(1.,0.,0.));
#6767=CARTESIAN_POINT('',(0.,0.,0.));
#6768=CARTESIAN_POINT('Origin',(1.18440385848747,0.,1.18440385848747));
#6769=CARTESIAN_POINT('',(0.846804978391753,-0.07938,1.40825612658882));
#6770=CARTESIAN_POINT('',(1.40825612658882,-0.07938,0.846804978391754));
#6771=CARTESIAN_POINT('Ctrl Pts',(0.846804978391752,-0.0793800000000001,
1.40825612658882));
#6772=CARTESIAN_POINT('Ctrl Pts',(0.854205272175554,-0.123401821157026,
1.40380622184538));
#6773=CARTESIAN_POINT('Ctrl Pts',(0.867957148219441,-0.166543350814306,
1.39550172959303));
#6774=CARTESIAN_POINT('Ctrl Pts',(0.902193646979982,-0.237231147975234,
1.3735491215176));
#6775=CARTESIAN_POINT('Ctrl Pts',(0.920778333482564,-0.266264900654909,
1.36127834356734));
#6776=CARTESIAN_POINT('Ctrl Pts',(0.962485392528369,-0.317195968905306,
1.33211611256184));
#6777=CARTESIAN_POINT('Ctrl Pts',(0.985600426557816,-0.33909093068465,1.31521005565926));
#6778=CARTESIAN_POINT('Ctrl Pts',(1.03253285680459,-0.373586846396559,1.27866649102984));
#6779=CARTESIAN_POINT('Ctrl Pts',(1.05871835910697,-0.388086240756494,1.25722555095714));
#6780=CARTESIAN_POINT('Ctrl Pts',(1.11153475808518,-0.407068917407805,1.2107812086231));
#6781=CARTESIAN_POINT('Ctrl Pts',(1.13814686046673,-0.411552957311693,1.18575674747573));
#6782=CARTESIAN_POINT('Ctrl Pts',(1.18575674747573,-0.411552957311693,1.13814686046673));
#6783=CARTESIAN_POINT('Ctrl Pts',(1.2107812086231,-0.407068917407805,1.11153475808518));
#6784=CARTESIAN_POINT('Ctrl Pts',(1.25722555095713,-0.388086240756494,1.05871835910697));
#6785=CARTESIAN_POINT('Ctrl Pts',(1.27866649102984,-0.373586846396559,1.03253285680459));
#6786=CARTESIAN_POINT('Ctrl Pts',(1.31521005565926,-0.33909093068465,0.985600426557816));
#6787=CARTESIAN_POINT('Ctrl Pts',(1.33211611256184,-0.317195968905306,0.962485392528369));
#6788=CARTESIAN_POINT('Ctrl Pts',(1.36127834356734,-0.266264900654909,0.920778333482565));
#6789=CARTESIAN_POINT('Ctrl Pts',(1.3735491215176,-0.237231147975234,0.902193646979983));
#6790=CARTESIAN_POINT('Ctrl Pts',(1.39550172959303,-0.166543350814306,0.867957148219442));
#6791=CARTESIAN_POINT('Ctrl Pts',(1.40380622184538,-0.123401821157026,0.854205272175555));
#6792=CARTESIAN_POINT('Ctrl Pts',(1.40825612658882,-0.0793800000000001,
0.846804978391753));
#6793=CARTESIAN_POINT('',(0.886256117232623,-0.07938,1.45861320581289));
#6794=CARTESIAN_POINT('Origin',(1.18440385848747,-0.07938,1.18440385848747));
#6795=CARTESIAN_POINT('',(1.45861320581289,-0.07938,0.886256117232624));
#6796=CARTESIAN_POINT('Ctrl Pts',(1.45861320581289,-0.0793800000000001,
0.886256117232623));
#6797=CARTESIAN_POINT('Ctrl Pts',(1.45630208793976,-0.101649918886749,0.890059788636852));
#6798=CARTESIAN_POINT('Ctrl Pts',(1.45296717977858,-0.123823518623746,0.895520212222107));
#6799=CARTESIAN_POINT('Ctrl Pts',(1.43904931717599,-0.192480977588836,0.917859913453975));
#6800=CARTESIAN_POINT('Ctrl Pts',(1.4243271592157,-0.236152929235938,0.940896403863072));
#6801=CARTESIAN_POINT('Ctrl Pts',(1.39055359345152,-0.303141259068212,0.990027513266106));
#6802=CARTESIAN_POINT('Ctrl Pts',(1.36743459453896,-0.335108247315849,1.02199477007745));
#6803=CARTESIAN_POINT('Ctrl Pts',(1.32643091652006,-0.373243761060364,1.07446535104584));
#6804=CARTESIAN_POINT('Ctrl Pts',(1.30441816675528,-0.387888272594439,1.10126842659597));
#6805=CARTESIAN_POINT('Ctrl Pts',(1.25681160160691,-0.407041111792943,1.15530234155453));
#6806=CARTESIAN_POINT('Ctrl Pts',(1.23119764287622,-0.411552957311693,1.18251418313119));
#6807=CARTESIAN_POINT('Ctrl Pts',(1.18251418313119,-0.411552957311693,1.23119764287622));
#6808=CARTESIAN_POINT('Ctrl Pts',(1.15530234155453,-0.407041111792943,1.25681160160691));
#6809=CARTESIAN_POINT('Ctrl Pts',(1.10126842659597,-0.387888272594439,1.30441816675528));
#6810=CARTESIAN_POINT('Ctrl Pts',(1.07446535104584,-0.373243761060364,1.32643091652006));
#6811=CARTESIAN_POINT('Ctrl Pts',(1.02199477007745,-0.335108247315848,1.36743459453896));
#6812=CARTESIAN_POINT('Ctrl Pts',(0.990027513266105,-0.303141259068211,
1.39055359345152));
#6813=CARTESIAN_POINT('Ctrl Pts',(0.940896403863071,-0.236152929235937,
1.42432715921571));
#6814=CARTESIAN_POINT('Ctrl Pts',(0.917859913453974,-0.192480977588835,
1.43904931717599));
#6815=CARTESIAN_POINT('Ctrl Pts',(0.895520212222106,-0.123823518623745,
1.45296717977858));
#6816=CARTESIAN_POINT('Ctrl Pts',(0.890059788636851,-0.101649918886749,
1.45630208793976));
#6817=CARTESIAN_POINT('Ctrl Pts',(0.886256117232622,-0.0793800000000001,
1.45861320581289));
#6818=CARTESIAN_POINT('Origin',(1.18440385848747,-0.07938,1.18440385848747));
#6819=CARTESIAN_POINT('Origin',(0.,-0.27783,0.));
#6820=CARTESIAN_POINT('',(0.404717578595295,-0.07938,1.65807299932179));
#6821=CARTESIAN_POINT('Origin',(0.,-0.07938,0.));
#6822=CARTESIAN_POINT('',(-0.404717578595296,-0.07938,1.65807299932179));
#6823=CARTESIAN_POINT('Ctrl Pts',(0.404717578595296,-0.0793800000000001,
1.65807299932179));
#6824=CARTESIAN_POINT('Ctrl Pts',(0.400393769631747,-0.101649918886749,
1.65912839404491));
#6825=CARTESIAN_POINT('Ctrl Pts',(0.394174530911058,-0.123823518623745,
1.66063136041479));
#6826=CARTESIAN_POINT('Ctrl Pts',(0.368536561654407,-0.192480977588835,
1.66658649961961));
#6827=CARTESIAN_POINT('Ctrl Pts',(0.341837165343982,-0.236152929235937,
1.67246562047521));
#6828=CARTESIAN_POINT('Ctrl Pts',(0.283214707341173,-0.303141259068211,
1.68332504372461));
#6829=CARTESIAN_POINT('Ctrl Pts',(0.244262842368623,-0.335108247315849,
1.68958170688653));
#6830=CARTESIAN_POINT('Ctrl Pts',(0.178166559972324,-0.373243761060364,
1.69769003172132));
#6831=CARTESIAN_POINT('Ctrl Pts',(0.143648558862931,-0.387888272594439,
1.70107730356824));
#6832=CARTESIAN_POINT('Ctrl Pts',(0.0717778861362652,-0.407041111792943,
1.70562212620408));
#6833=CARTESIAN_POINT('Ctrl Pts',(0.0344244045173309,-0.411552957311693,
1.706752));
#6834=CARTESIAN_POINT('Ctrl Pts',(-0.0344244045173315,-0.411552957311693,
1.706752));
#6835=CARTESIAN_POINT('Ctrl Pts',(-0.0717778861362658,-0.407041111792943,
1.70562212620408));
#6836=CARTESIAN_POINT('Ctrl Pts',(-0.143648558862932,-0.387888272594439,
1.70107730356824));
#6837=CARTESIAN_POINT('Ctrl Pts',(-0.178166559972325,-0.373243761060364,
1.69769003172132));
#6838=CARTESIAN_POINT('Ctrl Pts',(-0.244262842368624,-0.335108247315849,
1.68958170688653));
#6839=CARTESIAN_POINT('Ctrl Pts',(-0.283214707341173,-0.303141259068212,
1.68332504372461));
#6840=CARTESIAN_POINT('Ctrl Pts',(-0.341837165343982,-0.236152929235937,
1.67246562047521));
#6841=CARTESIAN_POINT('Ctrl Pts',(-0.368536561654408,-0.192480977588835,
1.66658649961961));
#6842=CARTESIAN_POINT('Ctrl Pts',(-0.394174530911059,-0.123823518623745,
1.66063136041479));
#6843=CARTESIAN_POINT('Ctrl Pts',(-0.400393769631748,-0.101649918886749,
1.65912839404491));
#6844=CARTESIAN_POINT('Ctrl Pts',(-0.404717578595297,-0.0793800000000001,
1.65807299932179));
#6845=CARTESIAN_POINT('',(-0.886256117232624,-0.07938,1.45861320581289));
#6846=CARTESIAN_POINT('Origin',(0.,-0.07938,0.));
#6847=CARTESIAN_POINT('',(-1.45861320581289,-0.07938,0.886256117232623));
#6848=CARTESIAN_POINT('Ctrl Pts',(-0.886256117232623,-0.0793800000000001,
1.45861320581289));
#6849=CARTESIAN_POINT('Ctrl Pts',(-0.890059788636852,-0.101649918886749,
1.45630208793976));
#6850=CARTESIAN_POINT('Ctrl Pts',(-0.895520212222106,-0.123823518623745,
1.45296717977858));
#6851=CARTESIAN_POINT('Ctrl Pts',(-0.917859913453974,-0.192480977588835,
1.43904931717599));
#6852=CARTESIAN_POINT('Ctrl Pts',(-0.940896403863071,-0.236152929235937,
1.4243271592157));
#6853=CARTESIAN_POINT('Ctrl Pts',(-0.990027513266105,-0.303141259068211,
1.39055359345152));
#6854=CARTESIAN_POINT('Ctrl Pts',(-1.02199477007745,-0.335108247315848,
1.36743459453896));
#6855=CARTESIAN_POINT('Ctrl Pts',(-1.07446535104584,-0.373243761060364,
1.32643091652006));
#6856=CARTESIAN_POINT('Ctrl Pts',(-1.10126842659597,-0.387888272594439,
1.30441816675528));
#6857=CARTESIAN_POINT('Ctrl Pts',(-1.15530234155453,-0.407041111792943,
1.25681160160691));
#6858=CARTESIAN_POINT('Ctrl Pts',(-1.18251418313119,-0.411552957311693,
1.23119764287622));
#6859=CARTESIAN_POINT('Ctrl Pts',(-1.23119764287622,-0.411552957311693,
1.18251418313119));
#6860=CARTESIAN_POINT('Ctrl Pts',(-1.25681160160691,-0.407041111792943,
1.15530234155453));
#6861=CARTESIAN_POINT('Ctrl Pts',(-1.30441816675528,-0.387888272594439,
1.10126842659597));
#6862=CARTESIAN_POINT('Ctrl Pts',(-1.32643091652006,-0.373243761060365,
1.07446535104584));
#6863=CARTESIAN_POINT('Ctrl Pts',(-1.36743459453896,-0.335108247315849,
1.02199477007745));
#6864=CARTESIAN_POINT('Ctrl Pts',(-1.39055359345152,-0.303141259068212,
0.990027513266106));
#6865=CARTESIAN_POINT('Ctrl Pts',(-1.4243271592157,-0.236152929235938,0.940896403863071));
#6866=CARTESIAN_POINT('Ctrl Pts',(-1.43904931717599,-0.192480977588836,
0.917859913453974));
#6867=CARTESIAN_POINT('Ctrl Pts',(-1.45296717977858,-0.123823518623746,
0.895520212222106));
#6868=CARTESIAN_POINT('Ctrl Pts',(-1.45630208793976,-0.101649918886749,
0.890059788636852));
#6869=CARTESIAN_POINT('Ctrl Pts',(-1.45861320581289,-0.0793800000000001,
0.886256117232623));
#6870=CARTESIAN_POINT('',(-1.65807299932179,-0.07938,0.404717578595295));
#6871=CARTESIAN_POINT('Origin',(0.,-0.07938,0.));
#6872=CARTESIAN_POINT('',(-1.706752,-0.411552957311693,2.08591827245526E-16));
#6873=CARTESIAN_POINT('Ctrl Pts',(-1.65807299932179,-0.0793800000000001,
0.404717578595296));
#6874=CARTESIAN_POINT('Ctrl Pts',(-1.65912839404491,-0.101649918886749,
0.400393769631747));
#6875=CARTESIAN_POINT('Ctrl Pts',(-1.66063136041479,-0.123823518623745,
0.394174530911058));
#6876=CARTESIAN_POINT('Ctrl Pts',(-1.66658649961961,-0.192480977588835,
0.368536561654407));
#6877=CARTESIAN_POINT('Ctrl Pts',(-1.67246562047521,-0.236152929235937,
0.341837165343982));
#6878=CARTESIAN_POINT('Ctrl Pts',(-1.68332504372461,-0.303141259068211,
0.283214707341173));
#6879=CARTESIAN_POINT('Ctrl Pts',(-1.68958170688653,-0.335108247315848,
0.244262842368623));
#6880=CARTESIAN_POINT('Ctrl Pts',(-1.69769003172132,-0.373243761060364,
0.178166559972324));
#6881=CARTESIAN_POINT('Ctrl Pts',(-1.70107730356824,-0.387888272594439,
0.143648558862931));
#6882=CARTESIAN_POINT('Ctrl Pts',(-1.70562212620408,-0.407041111792943,
0.0717778861362656));
#6883=CARTESIAN_POINT('Ctrl Pts',(-1.706752,-0.411552957311693,0.0344244045173313));
#6884=CARTESIAN_POINT('Ctrl Pts',(-1.706752,-0.411552957311693,2.08166817117217E-16));
#6885=CARTESIAN_POINT('',(-1.706752,-0.47628,2.09016837373834E-16));
#6886=CARTESIAN_POINT('',(-1.706752,-0.27783,2.09016837373834E-16));
#6887=CARTESIAN_POINT('Origin',(0.,-0.47628,0.));
#6888=CARTESIAN_POINT('',(-1.65807299932179,-0.07938,-0.404717578595296));
#6889=CARTESIAN_POINT('Ctrl Pts',(-1.706752,-0.411552957311693,2.0122792321331E-16));
#6890=CARTESIAN_POINT('Ctrl Pts',(-1.706752,-0.411552957311693,-0.0344244045173309));
#6891=CARTESIAN_POINT('Ctrl Pts',(-1.70562212620408,-0.407041111792943,
-0.0717778861362652));
#6892=CARTESIAN_POINT('Ctrl Pts',(-1.70107730356824,-0.387888272594439,
-0.143648558862931));
#6893=CARTESIAN_POINT('Ctrl Pts',(-1.69769003172132,-0.373243761060365,
-0.178166559972324));
#6894=CARTESIAN_POINT('Ctrl Pts',(-1.68958170688653,-0.335108247315849,
-0.244262842368623));
#6895=CARTESIAN_POINT('Ctrl Pts',(-1.68332504372461,-0.303141259068212,
-0.283214707341173));
#6896=CARTESIAN_POINT('Ctrl Pts',(-1.67246562047521,-0.236152929235938,
-0.341837165343982));
#6897=CARTESIAN_POINT('Ctrl Pts',(-1.66658649961961,-0.192480977588836,
-0.368536561654407));
#6898=CARTESIAN_POINT('Ctrl Pts',(-1.66063136041479,-0.123823518623745,
-0.394174530911059));
#6899=CARTESIAN_POINT('Ctrl Pts',(-1.65912839404491,-0.101649918886749,
-0.400393769631748));
#6900=CARTESIAN_POINT('Ctrl Pts',(-1.65807299932179,-0.0793800000000001,
-0.404717578595296));
#6901=CARTESIAN_POINT('',(-1.45861320581289,-0.07938,-0.886256117232623));
#6902=CARTESIAN_POINT('Origin',(0.,-0.07938,0.));
#6903=CARTESIAN_POINT('',(-0.886256117232623,-0.07938,-1.45861320581289));
#6904=CARTESIAN_POINT('Ctrl Pts',(-1.45861320581289,-0.0793800000000001,
-0.886256117232623));
#6905=CARTESIAN_POINT('Ctrl Pts',(-1.45630208793976,-0.101649918886749,
-0.890059788636852));
#6906=CARTESIAN_POINT('Ctrl Pts',(-1.45296717977858,-0.123823518623745,
-0.895520212222106));
#6907=CARTESIAN_POINT('Ctrl Pts',(-1.43904931717599,-0.192480977588835,
-0.917859913453974));
#6908=CARTESIAN_POINT('Ctrl Pts',(-1.4243271592157,-0.236152929235937,-0.940896403863072));
#6909=CARTESIAN_POINT('Ctrl Pts',(-1.39055359345152,-0.303141259068212,
-0.990027513266106));
#6910=CARTESIAN_POINT('Ctrl Pts',(-1.36743459453896,-0.335108247315849,
-1.02199477007745));
#6911=CARTESIAN_POINT('Ctrl Pts',(-1.32643091652006,-0.373243761060364,
-1.07446535104584));
#6912=CARTESIAN_POINT('Ctrl Pts',(-1.30441816675528,-0.387888272594439,
-1.10126842659597));
#6913=CARTESIAN_POINT('Ctrl Pts',(-1.25681160160691,-0.407041111792943,
-1.15530234155453));
#6914=CARTESIAN_POINT('Ctrl Pts',(-1.23119764287622,-0.411552957311693,
-1.18251418313119));
#6915=CARTESIAN_POINT('Ctrl Pts',(-1.18251418313119,-0.411552957311693,
-1.23119764287622));
#6916=CARTESIAN_POINT('Ctrl Pts',(-1.15530234155453,-0.407041111792943,
-1.25681160160691));
#6917=CARTESIAN_POINT('Ctrl Pts',(-1.10126842659597,-0.387888272594439,
-1.30441816675528));
#6918=CARTESIAN_POINT('Ctrl Pts',(-1.07446535104584,-0.373243761060364,
-1.32643091652006));
#6919=CARTESIAN_POINT('Ctrl Pts',(-1.02199477007745,-0.335108247315848,
-1.36743459453896));
#6920=CARTESIAN_POINT('Ctrl Pts',(-0.990027513266105,-0.303141259068211,
-1.39055359345152));
#6921=CARTESIAN_POINT('Ctrl Pts',(-0.940896403863071,-0.236152929235936,
-1.42432715921571));
#6922=CARTESIAN_POINT('Ctrl Pts',(-0.917859913453974,-0.192480977588835,
-1.43904931717599));
#6923=CARTESIAN_POINT('Ctrl Pts',(-0.895520212222106,-0.123823518623745,
-1.45296717977858));
#6924=CARTESIAN_POINT('Ctrl Pts',(-0.890059788636851,-0.101649918886749,
-1.45630208793976));
#6925=CARTESIAN_POINT('Ctrl Pts',(-0.886256117232623,-0.0793800000000001,
-1.45861320581289));
#6926=CARTESIAN_POINT('',(-0.404717578595295,-0.07938,-1.65807299932179));
#6927=CARTESIAN_POINT('Origin',(0.,-0.07938,0.));
#6928=CARTESIAN_POINT('',(0.404717578595296,-0.07938,-1.65807299932179));
#6929=CARTESIAN_POINT('Ctrl Pts',(-0.404717578595296,-0.0793800000000001,
-1.65807299932179));
#6930=CARTESIAN_POINT('Ctrl Pts',(-0.400393769631747,-0.101649918886749,
-1.65912839404491));
#6931=CARTESIAN_POINT('Ctrl Pts',(-0.394174530911058,-0.123823518623746,
-1.66063136041479));
#6932=CARTESIAN_POINT('Ctrl Pts',(-0.368536561654407,-0.192480977588836,
-1.66658649961961));
#6933=CARTESIAN_POINT('Ctrl Pts',(-0.341837165343982,-0.236152929235938,
-1.67246562047521));
#6934=CARTESIAN_POINT('Ctrl Pts',(-0.283214707341173,-0.303141259068212,
-1.68332504372461));
#6935=CARTESIAN_POINT('Ctrl Pts',(-0.244262842368623,-0.335108247315849,
-1.68958170688653));
#6936=CARTESIAN_POINT('Ctrl Pts',(-0.178166559972324,-0.373243761060364,
-1.69769003172132));
#6937=CARTESIAN_POINT('Ctrl Pts',(-0.143648558862931,-0.387888272594439,
-1.70107730356824));
#6938=CARTESIAN_POINT('Ctrl Pts',(-0.0717778861362653,-0.407041111792943,
-1.70562212620408));
#6939=CARTESIAN_POINT('Ctrl Pts',(-0.034424404517331,-0.411552957311693,
-1.706752));
#6940=CARTESIAN_POINT('Ctrl Pts',(0.0344244045173312,-0.411552957311693,
-1.706752));
#6941=CARTESIAN_POINT('Ctrl Pts',(0.0717778861362655,-0.407041111792943,
-1.70562212620408));
#6942=CARTESIAN_POINT('Ctrl Pts',(0.143648558862931,-0.387888272594439,
-1.70107730356824));
#6943=CARTESIAN_POINT('Ctrl Pts',(0.178166559972324,-0.373243761060364,
-1.69769003172132));
#6944=CARTESIAN_POINT('Ctrl Pts',(0.244262842368623,-0.335108247315849,
-1.68958170688653));
#6945=CARTESIAN_POINT('Ctrl Pts',(0.283214707341173,-0.303141259068212,
-1.68332504372461));
#6946=CARTESIAN_POINT('Ctrl Pts',(0.341837165343982,-0.236152929235937,
-1.67246562047521));
#6947=CARTESIAN_POINT('Ctrl Pts',(0.368536561654407,-0.192480977588835,
-1.66658649961961));
#6948=CARTESIAN_POINT('Ctrl Pts',(0.394174530911059,-0.123823518623745,
-1.66063136041479));
#6949=CARTESIAN_POINT('Ctrl Pts',(0.400393769631748,-0.101649918886749,
-1.65912839404491));
#6950=CARTESIAN_POINT('Ctrl Pts',(0.404717578595296,-0.0793800000000001,
-1.65807299932179));
#6951=CARTESIAN_POINT('',(0.886256117232623,-0.07938,-1.45861320581289));
#6952=CARTESIAN_POINT('Origin',(0.,-0.07938,0.));
#6953=CARTESIAN_POINT('',(1.45861320581289,-0.07938,-0.886256117232623));
#6954=CARTESIAN_POINT('Ctrl Pts',(0.886256117232623,-0.0793800000000001,
-1.45861320581289));
#6955=CARTESIAN_POINT('Ctrl Pts',(0.890059788636852,-0.101649918886749,
-1.45630208793976));
#6956=CARTESIAN_POINT('Ctrl Pts',(0.895520212222106,-0.123823518623745,
-1.45296717977858));
#6957=CARTESIAN_POINT('Ctrl Pts',(0.917859913453974,-0.192480977588835,
-1.43904931717599));
#6958=CARTESIAN_POINT('Ctrl Pts',(0.940896403863072,-0.236152929235937,
-1.4243271592157));
#6959=CARTESIAN_POINT('Ctrl Pts',(0.990027513266106,-0.303141259068211,
-1.39055359345152));
#6960=CARTESIAN_POINT('Ctrl Pts',(1.02199477007745,-0.335108247315849,-1.36743459453896));
#6961=CARTESIAN_POINT('Ctrl Pts',(1.07446535104584,-0.373243761060364,-1.32643091652006));
#6962=CARTESIAN_POINT('Ctrl Pts',(1.10126842659597,-0.387888272594439,-1.30441816675528));
#6963=CARTESIAN_POINT('Ctrl Pts',(1.15530234155453,-0.407041111792943,-1.25681160160691));
#6964=CARTESIAN_POINT('Ctrl Pts',(1.18251418313119,-0.411552957311693,-1.23119764287622));
#6965=CARTESIAN_POINT('Ctrl Pts',(1.23119764287622,-0.411552957311693,-1.18251418313119));
#6966=CARTESIAN_POINT('Ctrl Pts',(1.25681160160691,-0.407041111792943,-1.15530234155453));
#6967=CARTESIAN_POINT('Ctrl Pts',(1.30441816675528,-0.387888272594439,-1.10126842659597));
#6968=CARTESIAN_POINT('Ctrl Pts',(1.32643091652006,-0.373243761060364,-1.07446535104584));
#6969=CARTESIAN_POINT('Ctrl Pts',(1.36743459453896,-0.335108247315849,-1.02199477007745));
#6970=CARTESIAN_POINT('Ctrl Pts',(1.39055359345152,-0.303141259068212,-0.990027513266105));
#6971=CARTESIAN_POINT('Ctrl Pts',(1.4243271592157,-0.236152929235937,-0.940896403863071));
#6972=CARTESIAN_POINT('Ctrl Pts',(1.43904931717599,-0.192480977588835,-0.917859913453974));
#6973=CARTESIAN_POINT('Ctrl Pts',(1.45296717977858,-0.123823518623745,-0.895520212222106));
#6974=CARTESIAN_POINT('Ctrl Pts',(1.45630208793976,-0.101649918886749,-0.890059788636852));
#6975=CARTESIAN_POINT('Ctrl Pts',(1.45861320581289,-0.0793800000000001,
-0.886256117232623));
#6976=CARTESIAN_POINT('',(1.65807299932179,-0.07938,-0.404717578595296));
#6977=CARTESIAN_POINT('Origin',(0.,-0.07938,0.));
#6978=CARTESIAN_POINT('',(1.65807299932179,-0.07938,0.404717578595296));
#6979=CARTESIAN_POINT('Ctrl Pts',(1.65807299932179,-0.0793800000000001,
-0.404717578595296));
#6980=CARTESIAN_POINT('Ctrl Pts',(1.65912839404491,-0.101649918886749,-0.400393769631747));
#6981=CARTESIAN_POINT('Ctrl Pts',(1.66063136041479,-0.123823518623745,-0.394174530911058));
#6982=CARTESIAN_POINT('Ctrl Pts',(1.66658649961961,-0.192480977588835,-0.368536561654407));
#6983=CARTESIAN_POINT('Ctrl Pts',(1.67246562047521,-0.236152929235937,-0.341837165343982));
#6984=CARTESIAN_POINT('Ctrl Pts',(1.68332504372461,-0.303141259068212,-0.283214707341173));
#6985=CARTESIAN_POINT('Ctrl Pts',(1.68958170688653,-0.335108247315849,-0.244262842368623));
#6986=CARTESIAN_POINT('Ctrl Pts',(1.69769003172132,-0.373243761060364,-0.178166559972324));
#6987=CARTESIAN_POINT('Ctrl Pts',(1.70107730356824,-0.387888272594439,-0.143648558862931));
#6988=CARTESIAN_POINT('Ctrl Pts',(1.70562212620408,-0.407041111792943,-0.0717778861362655));
#6989=CARTESIAN_POINT('Ctrl Pts',(1.706752,-0.411552957311693,-0.0344244045173312));
#6990=CARTESIAN_POINT('Ctrl Pts',(1.706752,-0.411552957311693,0.0344244045173312));
#6991=CARTESIAN_POINT('Ctrl Pts',(1.70562212620408,-0.407041111792943,0.0717778861362655));
#6992=CARTESIAN_POINT('Ctrl Pts',(1.70107730356824,-0.387888272594439,0.143648558862931));
#6993=CARTESIAN_POINT('Ctrl Pts',(1.69769003172132,-0.373243761060364,0.178166559972324));
#6994=CARTESIAN_POINT('Ctrl Pts',(1.68958170688653,-0.335108247315849,0.244262842368623));
#6995=CARTESIAN_POINT('Ctrl Pts',(1.68332504372461,-0.303141259068212,0.283214707341173));
#6996=CARTESIAN_POINT('Ctrl Pts',(1.67246562047521,-0.236152929235937,0.341837165343982));
#6997=CARTESIAN_POINT('Ctrl Pts',(1.66658649961961,-0.192480977588835,0.368536561654407));
#6998=CARTESIAN_POINT('Ctrl Pts',(1.66063136041479,-0.123823518623745,0.394174530911058));
#6999=CARTESIAN_POINT('Ctrl Pts',(1.65912839404491,-0.101649918886749,0.400393769631747));
#7000=CARTESIAN_POINT('Ctrl Pts',(1.65807299932179,-0.0793800000000001,
0.404717578595296));
#7001=CARTESIAN_POINT('Origin',(0.,-0.07938,0.));
#7002=CARTESIAN_POINT('Origin',(0.,-0.07938,0.));
#7003=CARTESIAN_POINT('',(0.397005914195118,-0.07938,1.59456899932179));
#7004=CARTESIAN_POINT('Origin',(0.,-0.07938,0.));
#7005=CARTESIAN_POINT('Origin',(-3.33066907387547E-16,-0.07938,1.675));
#7006=CARTESIAN_POINT('Origin',(-3.33066907387547E-16,0.,1.675));
#7007=CARTESIAN_POINT('',(-0.397005914195118,-0.07938,1.59456899932179));
#7008=CARTESIAN_POINT('Ctrl Pts',(-0.397005914195119,-0.0793800000000001,
1.59456899932179));
#7009=CARTESIAN_POINT('Ctrl Pts',(-0.3886265584581,-0.123401821157026,1.59665523941937));
#7010=CARTESIAN_POINT('Ctrl Pts',(-0.373030350867485,-0.166543350814306,
1.60050712143809));
#7011=CARTESIAN_POINT('Ctrl Pts',(-0.333298652394954,-0.237231147975234,
1.60919314384089));
#7012=CARTESIAN_POINT('Ctrl Pts',(-0.311480544243687,-0.266264900654909,
1.61365775139403));
#7013=CARTESIAN_POINT('Ctrl Pts',(-0.261368388670537,-0.317195968905306,
1.62252828437015));
#7014=CARTESIAN_POINT('Ctrl Pts',(-0.233069203882014,-0.33909093068465,
1.62691869420078));
#7015=CARTESIAN_POINT('Ctrl Pts',(-0.174042761838764,-0.373586846396559,
1.63426473152765));
#7016=CARTESIAN_POINT('Ctrl Pts',(-0.14036578147155,-0.388086240756494,
1.63761964365402));
#7017=CARTESIAN_POINT('Ctrl Pts',(-0.0701778381840615,-0.407068917407805,
1.64212536811722));
#7018=CARTESIAN_POINT('Ctrl Pts',(-0.0336652739555918,-0.411552957311693,
1.643248));
#7019=CARTESIAN_POINT('Ctrl Pts',(0.0336652739555913,-0.411552957311693,
1.643248));
#7020=CARTESIAN_POINT('Ctrl Pts',(0.070177838184061,-0.407068917407805,
1.64212536811722));
#7021=CARTESIAN_POINT('Ctrl Pts',(0.140365781471549,-0.388086240756494,
1.63761964365402));
#7022=CARTESIAN_POINT('Ctrl Pts',(0.174042761838763,-0.373586846396559,
1.63426473152765));
#7023=CARTESIAN_POINT('Ctrl Pts',(0.233069203882014,-0.33909093068465,1.62691869420078));
#7024=CARTESIAN_POINT('Ctrl Pts',(0.261368388670536,-0.317195968905306,
1.62252828437015));
#7025=CARTESIAN_POINT('Ctrl Pts',(0.311480544243686,-0.266264900654908,
1.61365775139403));
#7026=CARTESIAN_POINT('Ctrl Pts',(0.333298652394954,-0.237231147975234,
1.60919314384089));
#7027=CARTESIAN_POINT('Ctrl Pts',(0.373030350867484,-0.166543350814306,
1.60050712143809));
#7028=CARTESIAN_POINT('Ctrl Pts',(0.388626558458099,-0.123401821157026,
1.59665523941937));
#7029=CARTESIAN_POINT('Ctrl Pts',(0.397005914195118,-0.07938,1.59456899932179));
#7030=CARTESIAN_POINT('Origin',(-3.33066907387547E-16,-0.07938,1.675));
#7031=CARTESIAN_POINT('Origin',(0.,-0.07938,0.));
#7032=CARTESIAN_POINT('',(-0.846804978391754,-0.07938,1.40825612658882));
#7033=CARTESIAN_POINT('Origin',(0.,-0.07938,0.));
#7034=CARTESIAN_POINT('Origin',(-1.18440385848747,-0.07938,1.18440385848747));
#7035=CARTESIAN_POINT('Origin',(-1.18440385848747,0.,1.18440385848747));
#7036=CARTESIAN_POINT('',(-1.40825612658882,-0.07938,0.846804978391753));
#7037=CARTESIAN_POINT('Ctrl Pts',(-1.40825612658882,-0.0793800000000001,
0.846804978391753));
#7038=CARTESIAN_POINT('Ctrl Pts',(-1.40380622184538,-0.123401821157026,
0.854205272175555));
#7039=CARTESIAN_POINT('Ctrl Pts',(-1.39550172959303,-0.166543350814306,
0.867957148219442));
#7040=CARTESIAN_POINT('Ctrl Pts',(-1.3735491215176,-0.237231147975235,0.902193646979983));
#7041=CARTESIAN_POINT('Ctrl Pts',(-1.36127834356734,-0.266264900654909,
0.920778333482565));
#7042=CARTESIAN_POINT('Ctrl Pts',(-1.33211611256184,-0.317195968905306,
0.962485392528369));
#7043=CARTESIAN_POINT('Ctrl Pts',(-1.31521005565926,-0.339090930684651,
0.985600426557816));
#7044=CARTESIAN_POINT('Ctrl Pts',(-1.27866649102984,-0.373586846396559,
1.03253285680459));
#7045=CARTESIAN_POINT('Ctrl Pts',(-1.25722555095714,-0.388086240756494,
1.05871835910697));
#7046=CARTESIAN_POINT('Ctrl Pts',(-1.2107812086231,-0.407068917407805,1.11153475808518));
#7047=CARTESIAN_POINT('Ctrl Pts',(-1.18575674747573,-0.411552957311693,
1.13814686046673));
#7048=CARTESIAN_POINT('Ctrl Pts',(-1.13814686046673,-0.411552957311693,
1.18575674747573));
#7049=CARTESIAN_POINT('Ctrl Pts',(-1.11153475808518,-0.407068917407805,
1.2107812086231));
#7050=CARTESIAN_POINT('Ctrl Pts',(-1.05871835910697,-0.388086240756494,
1.25722555095714));
#7051=CARTESIAN_POINT('Ctrl Pts',(-1.03253285680459,-0.373586846396559,
1.27866649102984));
#7052=CARTESIAN_POINT('Ctrl Pts',(-0.985600426557816,-0.33909093068465,
1.31521005565926));
#7053=CARTESIAN_POINT('Ctrl Pts',(-0.962485392528369,-0.317195968905306,
1.33211611256184));
#7054=CARTESIAN_POINT('Ctrl Pts',(-0.920778333482565,-0.266264900654908,
1.36127834356734));
#7055=CARTESIAN_POINT('Ctrl Pts',(-0.902193646979983,-0.237231147975234,
1.3735491215176));
#7056=CARTESIAN_POINT('Ctrl Pts',(-0.867957148219442,-0.166543350814306,
1.39550172959303));
#7057=CARTESIAN_POINT('Ctrl Pts',(-0.854205272175555,-0.123401821157026,
1.40380622184538));
#7058=CARTESIAN_POINT('Ctrl Pts',(-0.846804978391753,-0.0793800000000001,
1.40825612658882));
#7059=CARTESIAN_POINT('Origin',(-1.18440385848747,-0.07938,1.18440385848747));
#7060=CARTESIAN_POINT('Origin',(0.,-0.07938,0.));
#7061=CARTESIAN_POINT('',(-1.59456899932179,-0.07938,0.397005914195118));
#7062=CARTESIAN_POINT('Origin',(0.,-0.07938,0.));
#7063=CARTESIAN_POINT('Origin',(-1.675,-0.07938,-2.22044604925031E-16));
#7064=CARTESIAN_POINT('Origin',(-1.675,0.,-2.22044604925031E-16));
#7065=CARTESIAN_POINT('',(-1.59456899932179,-0.07938,-0.397005914195118));
#7066=CARTESIAN_POINT('',(-1.643248,-0.411552957311693,3.47540551556327E-18));
#7067=CARTESIAN_POINT('Ctrl Pts',(-1.59456899932179,-0.0793800000000001,
-0.397005914195119));
#7068=CARTESIAN_POINT('Ctrl Pts',(-1.59665523941937,-0.123401821157026,
-0.388626558458099));
#7069=CARTESIAN_POINT('Ctrl Pts',(-1.60050712143809,-0.166543350814306,
-0.373030350867485));
#7070=CARTESIAN_POINT('Ctrl Pts',(-1.60919314384089,-0.237231147975234,
-0.333298652394954));
#7071=CARTESIAN_POINT('Ctrl Pts',(-1.61365775139403,-0.266264900654909,
-0.311480544243686));
#7072=CARTESIAN_POINT('Ctrl Pts',(-1.62252828437015,-0.317195968905306,
-0.261368388670537));
#7073=CARTESIAN_POINT('Ctrl Pts',(-1.62691869420078,-0.33909093068465,-0.233069203882014));
#7074=CARTESIAN_POINT('Ctrl Pts',(-1.63426473152765,-0.373586846396559,
-0.174042761838764));
#7075=CARTESIAN_POINT('Ctrl Pts',(-1.63761964365402,-0.388086240756494,
-0.140365781471549));
#7076=CARTESIAN_POINT('Ctrl Pts',(-1.64212536811722,-0.407068917407805,
-0.0701778381840614));
#7077=CARTESIAN_POINT('Ctrl Pts',(-1.643248,-0.411552957311693,-0.0336652739555917));
#7078=CARTESIAN_POINT('Ctrl Pts',(-1.643248,-0.411552957311693,-2.0122792321331E-16));
#7079=CARTESIAN_POINT('Origin',(-1.675,-0.07938,-2.22044604925031E-16));
#7080=CARTESIAN_POINT('Ctrl Pts',(-1.643248,-0.411552957311693,-1.94289029309402E-16));
#7081=CARTESIAN_POINT('Ctrl Pts',(-1.643248,-0.411552957311693,0.0336652739555913));
#7082=CARTESIAN_POINT('Ctrl Pts',(-1.64212536811722,-0.407068917407805,
0.0701778381840609));
#7083=CARTESIAN_POINT('Ctrl Pts',(-1.63761964365402,-0.388086240756494,
0.140365781471549));
#7084=CARTESIAN_POINT('Ctrl Pts',(-1.63426473152765,-0.373586846396559,
0.174042761838763));
#7085=CARTESIAN_POINT('Ctrl Pts',(-1.62691869420078,-0.33909093068465,0.233069203882014));
#7086=CARTESIAN_POINT('Ctrl Pts',(-1.62252828437015,-0.317195968905306,
0.261368388670536));
#7087=CARTESIAN_POINT('Ctrl Pts',(-1.61365775139403,-0.266264900654909,
0.311480544243686));
#7088=CARTESIAN_POINT('Ctrl Pts',(-1.60919314384089,-0.237231147975235,
0.333298652394954));
#7089=CARTESIAN_POINT('Ctrl Pts',(-1.60050712143809,-0.166543350814306,
0.373030350867484));
#7090=CARTESIAN_POINT('Ctrl Pts',(-1.59665523941937,-0.123401821157026,
0.388626558458099));
#7091=CARTESIAN_POINT('Ctrl Pts',(-1.59456899932179,-0.0793800000000001,
0.397005914195118));
#7092=CARTESIAN_POINT('Origin',(0.,-0.07938,0.));
#7093=CARTESIAN_POINT('',(-1.40825612658882,-0.07938,-0.846804978391753));
#7094=CARTESIAN_POINT('Origin',(0.,-0.07938,0.));
#7095=CARTESIAN_POINT('Origin',(-1.18440385848747,-0.07938,-1.18440385848747));
#7096=CARTESIAN_POINT('Origin',(-1.18440385848747,0.,-1.18440385848747));
#7097=CARTESIAN_POINT('',(-0.846804978391753,-0.07938,-1.40825612658882));
#7098=CARTESIAN_POINT('Ctrl Pts',(-0.846804978391753,-0.0793800000000001,
-1.40825612658882));
#7099=CARTESIAN_POINT('Ctrl Pts',(-0.854205272175555,-0.123401821157026,
-1.40380622184538));
#7100=CARTESIAN_POINT('Ctrl Pts',(-0.867957148219442,-0.166543350814306,
-1.39550172959303));
#7101=CARTESIAN_POINT('Ctrl Pts',(-0.902193646979982,-0.237231147975234,
-1.3735491215176));
#7102=CARTESIAN_POINT('Ctrl Pts',(-0.920778333482564,-0.266264900654908,
-1.36127834356734));
#7103=CARTESIAN_POINT('Ctrl Pts',(-0.962485392528368,-0.317195968905306,
-1.33211611256184));
#7104=CARTESIAN_POINT('Ctrl Pts',(-0.985600426557816,-0.33909093068465,
-1.31521005565926));
#7105=CARTESIAN_POINT('Ctrl Pts',(-1.03253285680459,-0.373586846396559,
-1.27866649102984));
#7106=CARTESIAN_POINT('Ctrl Pts',(-1.05871835910697,-0.388086240756494,
-1.25722555095714));
#7107=CARTESIAN_POINT('Ctrl Pts',(-1.11153475808518,-0.407068917407805,
-1.2107812086231));
#7108=CARTESIAN_POINT('Ctrl Pts',(-1.13814686046673,-0.411552957311693,
-1.18575674747573));
#7109=CARTESIAN_POINT('Ctrl Pts',(-1.18575674747573,-0.411552957311693,
-1.13814686046673));
#7110=CARTESIAN_POINT('Ctrl Pts',(-1.2107812086231,-0.407068917407805,-1.11153475808518));
#7111=CARTESIAN_POINT('Ctrl Pts',(-1.25722555095714,-0.388086240756494,
-1.05871835910697));
#7112=CARTESIAN_POINT('Ctrl Pts',(-1.27866649102984,-0.373586846396559,
-1.03253285680459));
#7113=CARTESIAN_POINT('Ctrl Pts',(-1.31521005565926,-0.33909093068465,-0.985600426557816));
#7114=CARTESIAN_POINT('Ctrl Pts',(-1.33211611256184,-0.317195968905306,
-0.962485392528369));
#7115=CARTESIAN_POINT('Ctrl Pts',(-1.36127834356734,-0.266264900654909,
-0.920778333482565));
#7116=CARTESIAN_POINT('Ctrl Pts',(-1.3735491215176,-0.237231147975234,-0.902193646979983));
#7117=CARTESIAN_POINT('Ctrl Pts',(-1.39550172959303,-0.166543350814306,
-0.867957148219442));
#7118=CARTESIAN_POINT('Ctrl Pts',(-1.40380622184538,-0.123401821157026,
-0.854205272175555));
#7119=CARTESIAN_POINT('Ctrl Pts',(-1.40825612658882,-0.07938,-0.846804978391753));
#7120=CARTESIAN_POINT('Origin',(-1.18440385848747,-0.07938,-1.18440385848747));
#7121=CARTESIAN_POINT('Origin',(0.,-0.07938,0.));
#7122=CARTESIAN_POINT('',(-0.397005914195118,-0.07938,-1.59456899932179));
#7123=CARTESIAN_POINT('Origin',(0.,-0.07938,0.));
#7124=CARTESIAN_POINT('Origin',(1.11022302462516E-16,-0.07938,-1.675));
#7125=CARTESIAN_POINT('Origin',(1.11022302462516E-16,0.,-1.675));
#7126=CARTESIAN_POINT('',(0.397005914195118,-0.07938,-1.59456899932179));
#7127=CARTESIAN_POINT('Ctrl Pts',(0.397005914195119,-0.0793800000000001,
-1.59456899932179));
#7128=CARTESIAN_POINT('Ctrl Pts',(0.388626558458099,-0.123401821157026,
-1.59665523941937));
#7129=CARTESIAN_POINT('Ctrl Pts',(0.373030350867485,-0.166543350814306,
-1.60050712143809));
#7130=CARTESIAN_POINT('Ctrl Pts',(0.333298652394954,-0.237231147975234,
-1.60919314384089));
#7131=CARTESIAN_POINT('Ctrl Pts',(0.311480544243686,-0.266264900654909,
-1.61365775139403));
#7132=CARTESIAN_POINT('Ctrl Pts',(0.261368388670537,-0.317195968905306,
-1.62252828437015));
#7133=CARTESIAN_POINT('Ctrl Pts',(0.233069203882014,-0.33909093068465,-1.62691869420078));
#7134=CARTESIAN_POINT('Ctrl Pts',(0.174042761838763,-0.373586846396559,
-1.63426473152765));
#7135=CARTESIAN_POINT('Ctrl Pts',(0.140365781471549,-0.388086240756494,
-1.63761964365402));
#7136=CARTESIAN_POINT('Ctrl Pts',(0.0701778381840612,-0.407068917407805,
-1.64212536811722));
#7137=CARTESIAN_POINT('Ctrl Pts',(0.0336652739555916,-0.411552957311693,
-1.643248));
#7138=CARTESIAN_POINT('Ctrl Pts',(-0.0336652739555915,-0.411552957311693,
-1.643248));
#7139=CARTESIAN_POINT('Ctrl Pts',(-0.0701778381840612,-0.407068917407805,
-1.64212536811722));
#7140=CARTESIAN_POINT('Ctrl Pts',(-0.140365781471549,-0.388086240756494,
-1.63761964365402));
#7141=CARTESIAN_POINT('Ctrl Pts',(-0.174042761838764,-0.373586846396559,
-1.63426473152765));
#7142=CARTESIAN_POINT('Ctrl Pts',(-0.233069203882014,-0.33909093068465,
-1.62691869420078));
#7143=CARTESIAN_POINT('Ctrl Pts',(-0.261368388670536,-0.317195968905306,
-1.62252828437015));
#7144=CARTESIAN_POINT('Ctrl Pts',(-0.311480544243686,-0.266264900654908,
-1.61365775139403));
#7145=CARTESIAN_POINT('Ctrl Pts',(-0.333298652394954,-0.237231147975234,
-1.60919314384089));
#7146=CARTESIAN_POINT('Ctrl Pts',(-0.373030350867485,-0.166543350814306,
-1.60050712143809));
#7147=CARTESIAN_POINT('Ctrl Pts',(-0.388626558458099,-0.123401821157026,
-1.59665523941937));
#7148=CARTESIAN_POINT('Ctrl Pts',(-0.397005914195118,-0.07938,-1.59456899932179));
#7149=CARTESIAN_POINT('Origin',(1.11022302462516E-16,-0.07938,-1.675));
#7150=CARTESIAN_POINT('Origin',(0.,-0.07938,0.));
#7151=CARTESIAN_POINT('',(0.846804978391753,-0.07938,-1.40825612658882));
#7152=CARTESIAN_POINT('Origin',(0.,-0.07938,0.));
#7153=CARTESIAN_POINT('Origin',(1.18440385848747,-0.07938,-1.18440385848747));
#7154=CARTESIAN_POINT('Origin',(1.18440385848747,0.,-1.18440385848747));
#7155=CARTESIAN_POINT('',(1.40825612658882,-0.07938,-0.846804978391753));
#7156=CARTESIAN_POINT('Ctrl Pts',(1.40825612658882,-0.0793800000000001,
-0.846804978391753));
#7157=CARTESIAN_POINT('Ctrl Pts',(1.40380622184538,-0.123401821157026,-0.854205272175555));
#7158=CARTESIAN_POINT('Ctrl Pts',(1.39550172959303,-0.166543350814306,-0.867957148219442));
#7159=CARTESIAN_POINT('Ctrl Pts',(1.3735491215176,-0.237231147975234,-0.902193646979983));
#7160=CARTESIAN_POINT('Ctrl Pts',(1.36127834356734,-0.266264900654908,-0.920778333482565));
#7161=CARTESIAN_POINT('Ctrl Pts',(1.33211611256184,-0.317195968905306,-0.962485392528369));
#7162=CARTESIAN_POINT('Ctrl Pts',(1.31521005565926,-0.33909093068465,-0.985600426557816));
#7163=CARTESIAN_POINT('Ctrl Pts',(1.27866649102984,-0.373586846396559,-1.03253285680459));
#7164=CARTESIAN_POINT('Ctrl Pts',(1.25722555095714,-0.388086240756494,-1.05871835910697));
#7165=CARTESIAN_POINT('Ctrl Pts',(1.2107812086231,-0.407068917407805,-1.11153475808518));
#7166=CARTESIAN_POINT('Ctrl Pts',(1.18575674747573,-0.411552957311693,-1.13814686046673));
#7167=CARTESIAN_POINT('Ctrl Pts',(1.13814686046673,-0.411552957311693,-1.18575674747573));
#7168=CARTESIAN_POINT('Ctrl Pts',(1.11153475808518,-0.407068917407805,-1.2107812086231));
#7169=CARTESIAN_POINT('Ctrl Pts',(1.05871835910697,-0.388086240756494,-1.25722555095714));
#7170=CARTESIAN_POINT('Ctrl Pts',(1.03253285680459,-0.373586846396559,-1.27866649102984));
#7171=CARTESIAN_POINT('Ctrl Pts',(0.985600426557816,-0.33909093068465,-1.31521005565926));
#7172=CARTESIAN_POINT('Ctrl Pts',(0.962485392528369,-0.317195968905306,
-1.33211611256184));
#7173=CARTESIAN_POINT('Ctrl Pts',(0.920778333482565,-0.266264900654909,
-1.36127834356734));
#7174=CARTESIAN_POINT('Ctrl Pts',(0.902193646979983,-0.237231147975234,
-1.3735491215176));
#7175=CARTESIAN_POINT('Ctrl Pts',(0.867957148219442,-0.166543350814306,
-1.39550172959303));
#7176=CARTESIAN_POINT('Ctrl Pts',(0.854205272175555,-0.123401821157026,
-1.40380622184538));
#7177=CARTESIAN_POINT('Ctrl Pts',(0.846804978391753,-0.0793800000000001,
-1.40825612658882));
#7178=CARTESIAN_POINT('Origin',(1.18440385848747,-0.07938,-1.18440385848747));
#7179=CARTESIAN_POINT('Origin',(0.,-0.27783,0.));
#7180=CARTESIAN_POINT('',(-1.643248,-0.47628,2.01239840340529E-16));
#7181=CARTESIAN_POINT('Origin',(0.,-0.47628,0.));
#7182=CARTESIAN_POINT('',(-1.643248,-0.27783,2.01239840340529E-16));
#7183=CARTESIAN_POINT('',(1.59456899932179,-0.07938,0.397005914195118));
#7184=CARTESIAN_POINT('Origin',(0.,-0.07938,0.));
#7185=CARTESIAN_POINT('',(1.59456899932179,-0.07938,-0.397005914195118));
#7186=CARTESIAN_POINT('Ctrl Pts',(1.59456899932179,-0.0793800000000001,
0.397005914195118));
#7187=CARTESIAN_POINT('Ctrl Pts',(1.59665523941937,-0.123401821157026,0.388626558458099));
#7188=CARTESIAN_POINT('Ctrl Pts',(1.60050712143809,-0.166543350814306,0.373030350867485));
#7189=CARTESIAN_POINT('Ctrl Pts',(1.60919314384089,-0.237231147975234,0.333298652394954));
#7190=CARTESIAN_POINT('Ctrl Pts',(1.61365775139403,-0.266264900654909,0.311480544243686));
#7191=CARTESIAN_POINT('Ctrl Pts',(1.62252828437015,-0.317195968905306,0.261368388670537));
#7192=CARTESIAN_POINT('Ctrl Pts',(1.62691869420078,-0.33909093068465,0.233069203882014));
#7193=CARTESIAN_POINT('Ctrl Pts',(1.63426473152765,-0.373586846396559,0.174042761838764));
#7194=CARTESIAN_POINT('Ctrl Pts',(1.63761964365402,-0.388086240756494,0.140365781471549));
#7195=CARTESIAN_POINT('Ctrl Pts',(1.64212536811722,-0.407068917407805,0.0701778381840612));
#7196=CARTESIAN_POINT('Ctrl Pts',(1.643248,-0.411552957311693,0.0336652739555916));
#7197=CARTESIAN_POINT('Ctrl Pts',(1.643248,-0.411552957311693,-0.0336652739555916));
#7198=CARTESIAN_POINT('Ctrl Pts',(1.64212536811722,-0.407068917407805,-0.0701778381840612));
#7199=CARTESIAN_POINT('Ctrl Pts',(1.63761964365402,-0.388086240756494,-0.140365781471549));
#7200=CARTESIAN_POINT('Ctrl Pts',(1.63426473152765,-0.373586846396559,-0.174042761838764));
#7201=CARTESIAN_POINT('Ctrl Pts',(1.62691869420078,-0.33909093068465,-0.233069203882014));
#7202=CARTESIAN_POINT('Ctrl Pts',(1.62252828437015,-0.317195968905306,-0.261368388670537));
#7203=CARTESIAN_POINT('Ctrl Pts',(1.61365775139403,-0.266264900654909,-0.311480544243686));
#7204=CARTESIAN_POINT('Ctrl Pts',(1.60919314384089,-0.237231147975234,-0.333298652394954));
#7205=CARTESIAN_POINT('Ctrl Pts',(1.60050712143809,-0.166543350814306,-0.373030350867485));
#7206=CARTESIAN_POINT('Ctrl Pts',(1.59665523941937,-0.123401821157026,-0.388626558458099));
#7207=CARTESIAN_POINT('Ctrl Pts',(1.59456899932179,-0.07938,-0.397005914195118));
#7208=CARTESIAN_POINT('Origin',(0.,-0.07938,0.));
#7209=CARTESIAN_POINT('Origin',(0.,-0.07938,0.));
#7210=CARTESIAN_POINT('Origin',(1.675,-0.07938,0.));
#7211=CARTESIAN_POINT('Origin',(1.675,0.,0.));
#7212=CARTESIAN_POINT('Origin',(1.675,-0.07938,0.));
#7213=CARTESIAN_POINT('Origin',(0.,-0.47628,0.));
#7214=CARTESIAN_POINT('Origin',(0.,-0.07938,0.));
#7834=UNCERTAINTY_MEASURE_WITH_UNIT(LENGTH_MEASURE(0.001),#7872,
'DISTANCE_ACCURACY_VALUE',
'Maximum model space distance between geometric entities at asserted c
onnectivities');
#7845=UNCERTAINTY_MEASURE_WITH_UNIT(LENGTH_MEASURE(0.001),#7872,
'DISTANCE_ACCURACY_VALUE',
'Maximum model space distance between geometric entities at asserted c
onnectivities');
#7860=(
GEOMETRIC_REPRESENTATION_CONTEXT(3)
GLOBAL_UNCERTAINTY_ASSIGNED_CONTEXT((#7834))
GLOBAL_UNIT_ASSIGNED_CONTEXT((#7872,#7874,#7875))
REPRESENTATION_CONTEXT('','3D')
);
#7871=(
GEOMETRIC_REPRESENTATION_CONTEXT(3)
GLOBAL_UNCERTAINTY_ASSIGNED_CONTEXT((#7845))
GLOBAL_UNIT_ASSIGNED_CONTEXT((#7872,#7874,#7875))
REPRESENTATION_CONTEXT('','3D')
);
#7872=(
LENGTH_UNIT()
NAMED_UNIT(*)
SI_UNIT(.CENTI.,.METRE.)
);
#7874=(
NAMED_UNIT(*)
PLANE_ANGLE_UNIT()
SI_UNIT($,.RADIAN.)
);
#7875=(
NAMED_UNIT(*)
SI_UNIT($,.STERADIAN.)
SOLID_ANGLE_UNIT()
);
#7890=SHAPE_DEFINITION_REPRESENTATION(#7915,#7976);
#7915=PRODUCT_DEFINITION_SHAPE('',$,#8002);
#7976=SHAPE_REPRESENTATION('',(#4613),#7860);
#7987=PRODUCT_DEFINITION_CONTEXT('part definition',#8064,'design');
#8002=PRODUCT_DEFINITION('Cage','Cage',#8027,#7987);
#8027=PRODUCT_DEFINITION_FORMATION('',$,#8080);
#8064=APPLICATION_CONTEXT(
'Core Data for Automotive Mechanical Design Process');
#8065=PRODUCT_CONTEXT('part definition',#8064,'mechanical');
#8080=PRODUCT('Cage','Cage','Cage',(#8065));
#8147=COLOUR_RGB('Grey',0.48,0.52,0.57);
#8148=FILL_AREA_STYLE_COLOUR('',#8147);
#8149=FILL_AREA_STYLE('',(#8148));
#8150=SURFACE_STYLE_FILL_AREA(#8149);
#8151=SURFACE_SIDE_STYLE('',(#8150));
#8152=SURFACE_STYLE_USAGE(.BOTH.,#8151);
#8153=PRESENTATION_STYLE_ASSIGNMENT((#8152));
ENDSEC;
END-ISO-10303-21;
